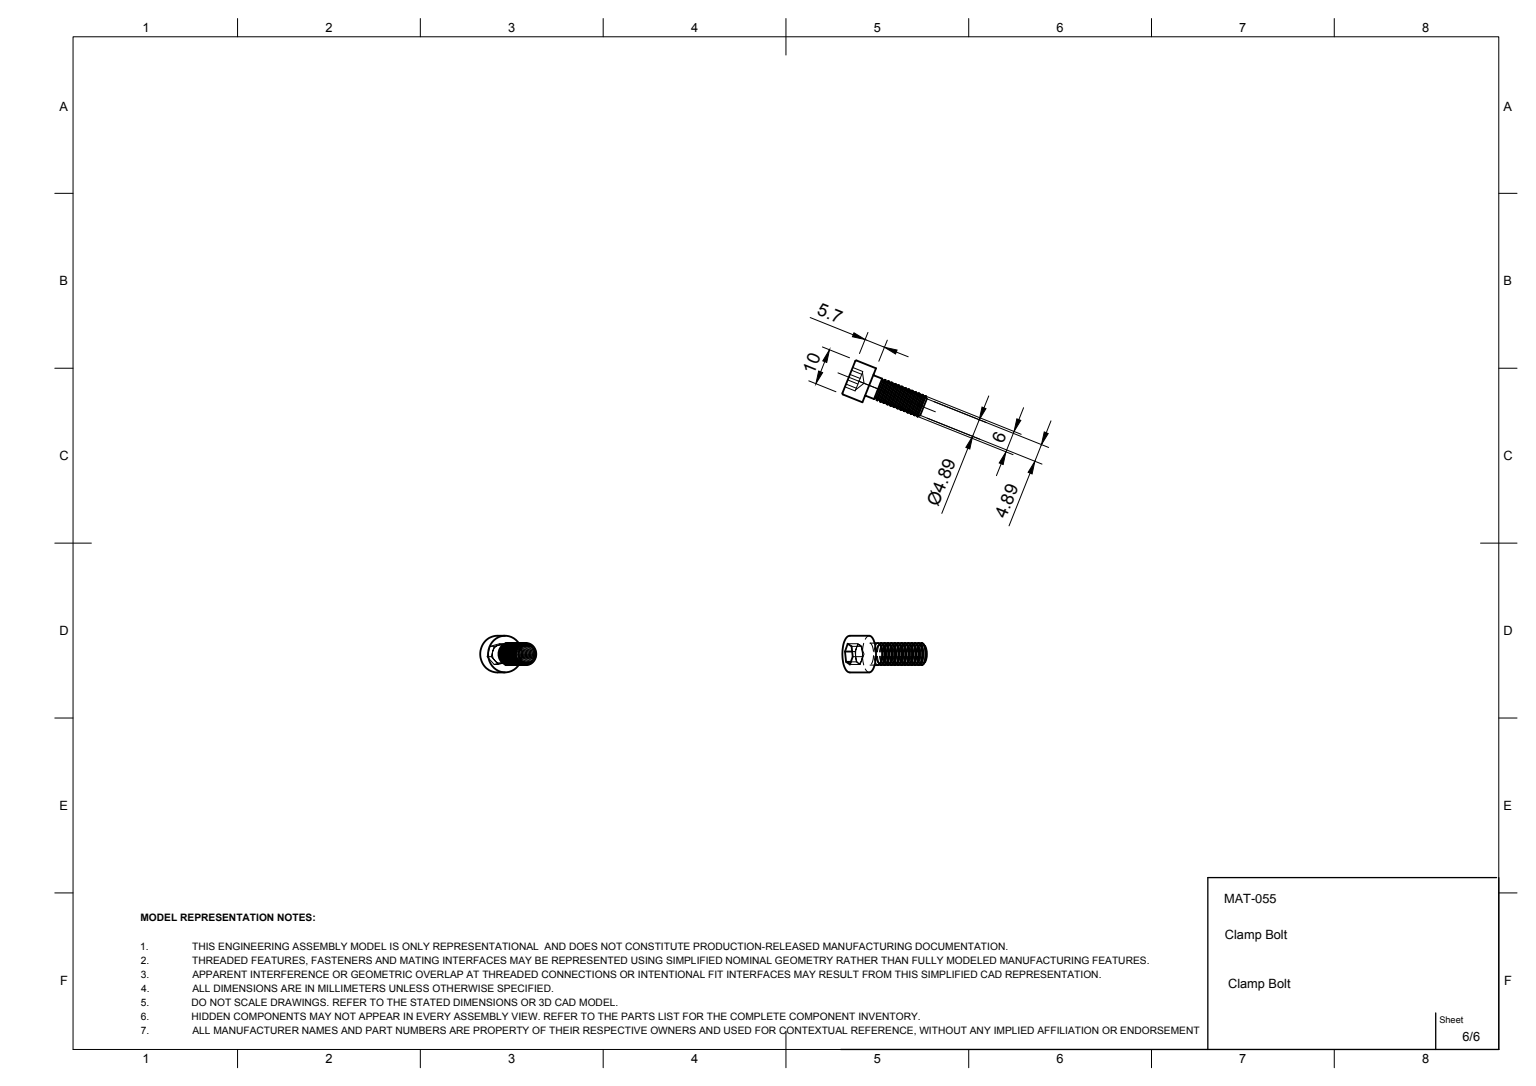
ISO-10303-21;
HEADER;
FILE_DESCRIPTION (('STEP AP214'),
    '1' );
FILE_NAME ('Clamp Bolt.step',
    '2026-10-30T09:41:00',
    ( '' ),
    ( '' ),
    'SwSTEP 2.0',
    'SolidWorks 2020',
    '' );
FILE_SCHEMA (( 'AUTOMOTIVE_DESIGN' ));
ENDSEC;

DATA;
#2=LINE ( 'NONE', #2744, #42488 ) ;
#10=FACE_OUTER_BOUND ( 'NONE', #7467, .T. ) ;
#27=AXIS2_PLACEMENT_3D ( 'NONE', #14609, #30094, #23021 ) ;
#30=LINE ( 'NONE', #27854, #4652 ) ;
#33=LINE ( 'NONE', #17589, #1125 ) ;
#38=DIRECTION ( 'NONE',  ( 0.9609149988134837450, -0.1028163501681639419, 0.2570431154366518145 ) ) ;
#58=DIRECTION ( 'NONE',  ( -0.000000000000000000, -0.9284778069183721172, -0.3713878862591650232 ) ) ;
#68=ORIENTED_EDGE ( 'NONE', *, *, #40399, .T. ) ;
#82=DIRECTION ( 'NONE',  ( 0.9609149988134837450, -0.1028163501681639419, 0.2570431154366518145 ) ) ;
#87=FACE_OUTER_BOUND ( 'NONE', #1657, .T. ) ;
#93=CARTESIAN_POINT ( 'NONE',  ( 71.02242295334774269, -99.02728775972636299, -55.91838671430374319 ) ) ;
#107=CARTESIAN_POINT ( 'NONE',  ( 69.36136150295220659, -60.18712133882883819, -34.17284023871924603 ) ) ;
#121=ORIENTED_EDGE ( 'NONE', *, *, #26803, .F. ) ;
#123=CIRCLE ( 'NONE', #28512, 2.445500000000004448 ) ;
#128=ORIENTED_EDGE ( 'NONE', *, *, #14994, .T. ) ;
#134=DIRECTION ( 'NONE',  ( -0.000000000000000000, -0.9284778069183718952, -0.3713878862591649677 ) ) ;
#135=CARTESIAN_POINT ( 'NONE',  ( 70.19189222814998175, -53.33815113939435548, -34.53808368179734600 ) ) ;
#167=CIRCLE ( 'NONE', #27232, 2.999999999999999556 ) ;
#169=AXIS2_PLACEMENT_3D ( 'NONE', #31050, #27866, #41779 ) ;
#179=EDGE_CURVE ( 'NONE', #39765, #40221, #19962, .T. ) ;
#191=CONICAL_SURFACE ( 'NONE', #23525, 2.999999999999999556, 0.9599310885968830309 ) ;
#193=VECTOR ( 'NONE', #10934, 1000.000000000000114 ) ;
#194=DIRECTION ( 'NONE',  ( -0.000000000000000000, -0.9284778069183721172, -0.3713878862591650232 ) ) ;
#216=EDGE_CURVE ( 'NONE', #33082, #17518, #26949, .T. ) ;
#219=VERTEX_POINT ( 'NONE', #5508 ) ;
#237=LINE ( 'NONE', #38306, #33556 ) ;
#238=EDGE_CURVE ( 'NONE', #18481, #11704, #33042, .T. ) ;
#251=DIRECTION ( 'NONE',  ( 0.2768435750659263284, 0.3568721902840676363, -0.8921882507333129819 ) ) ;
#252=CYLINDRICAL_SURFACE ( 'NONE', #41921, 3.000000000000001776 ) ;
#263=AXIS2_PLACEMENT_3D ( 'NONE', #1168, #7793, #17829 ) ;
#279=VERTEX_POINT ( 'NONE', #20785 ) ;
#280=AXIS2_PLACEMENT_3D ( 'NONE', #38645, #14273, #42543 ) ;
#302=LINE ( 'NONE', #3715, #30421 ) ;
#314=AXIS2_PLACEMENT_3D ( 'NONE', #35221, #3555, #37996 ) ;
#347=ORIENTED_EDGE ( 'NONE', *, *, #19251, .F. ) ;
#352=CARTESIAN_POINT ( 'NONE',  ( 67.84197459855160162, -60.15404070048191443, -37.99358876332483703 ) ) ;
#367=DIRECTION ( 'NONE',  ( -0.000000000000000000, -0.9284778069183718952, -0.3713878862591649677 ) ) ;
#384=CARTESIAN_POINT ( 'NONE',  ( 69.48536631248848039, -66.77523564985355620, -42.98127819198803934 ) ) ;
#406=CARTESIAN_POINT ( 'NONE',  ( 71.02242295334774269, -99.02728775972636299, -55.91838671430374319 ) ) ;
#416=CIRCLE ( 'NONE', #25919, 2.999999999999999556 ) ;
#429=DIRECTION ( 'NONE',  ( 1.387778780781445676E-17, -0.9284778069183720062, -0.3713878862591650232 ) ) ;
#435=FACE_OUTER_BOUND ( 'NONE', #25731, .T. ) ;
#454=DIRECTION ( 'NONE',  ( -0.2768435750659241079, -0.3568721902840695792, 0.8921882507333129819 ) ) ;
#482=DIRECTION ( 'NONE',  ( -0.2768435750659241079, -0.3568721902840695792, 0.8921882507333129819 ) ) ;
#487=DIRECTION ( 'NONE',  ( 0.9609149988134843001, -0.1028163501681632064, 0.2570431154366505933 ) ) ;
#495=EDGE_CURVE ( 'NONE', #29216, #38926, #30, .T. ) ;
#519=VECTOR ( 'NONE', #2199, 999.9999999999998863 ) ;
#545=ORIENTED_EDGE ( 'NONE', *, *, #32038, .F. ) ;
#572=AXIS2_PLACEMENT_3D ( 'NONE', #28197, #18381, #24548 ) ;
#587=EDGE_CURVE ( 'NONE', #3470, #34725, #44742, .T. ) ;
#591=DIRECTION ( 'NONE',  ( -0.000000000000000000, -0.9284778069183721172, -0.3713878862591650232 ) ) ;
#628=ORIENTED_EDGE ( 'NONE', *, *, #2447, .F. ) ;
#652=DIRECTION ( 'NONE',  ( 0.000000000000000000, 0.9284778069183720062, 0.3713878862591650232 ) ) ;
#663=ORIENTED_EDGE ( 'NONE', *, *, #32365, .T. ) ;
#730=ORIENTED_EDGE ( 'NONE', *, *, #26390, .T. ) ;
#731=AXIS2_PLACEMENT_3D ( 'NONE', #25829, #15568, #36529 ) ;
#769=LINE ( 'NONE', #29271, #10675 ) ;
#793=DIRECTION ( 'NONE',  ( -0.7871354856660162103, -0.4483307682966942709, -0.4235767337848251879 ) ) ;
#796=EDGE_CURVE ( 'NONE', #20803, #26292, #18485, .T. ) ;
#800=DIRECTION ( 'NONE',  ( 0.9609149988134837450, -0.1028163501681639419, 0.2570431154366518145 ) ) ;
#825=CONICAL_SURFACE ( 'NONE', #24153, 2.999999999999999556, 0.9599310885968830309 ) ;
#838=CARTESIAN_POINT ( 'NONE',  ( 70.19189222814998175, -62.26243369865490251, -38.10776559704283528 ) ) ;
#860=DIRECTION ( 'NONE',  ( -0.000000000000000000, -0.9284778069183718952, -0.3713878862591649677 ) ) ;
#871=FACE_OUTER_BOUND ( 'NONE', #3620, .T. ) ;
#876=LINE ( 'NONE', #14795, #14624 ) ;
#877=CARTESIAN_POINT ( 'NONE',  ( 70.19189222814998175, -59.83749578782295941, -37.13779888561150244 ) ) ;
#907=LINE ( 'NONE', #38753, #23410 ) ;
#909=AXIS2_PLACEMENT_3D ( 'NONE', #40106, #12526, #26200 ) ;
#910=DIRECTION ( 'NONE',  ( -0.000000000000000000, -0.9284778069183721172, -0.3713878862591650232 ) ) ;
#935=EDGE_CURVE ( 'NONE', #32198, #39653, #29454, .T. ) ;
#964=ORIENTED_EDGE ( 'NONE', *, *, #27844, .T. ) ;
#989=AXIS2_PLACEMENT_3D ( 'NONE', #41662, #38211, #6989 ) ;
#993=ORIENTED_EDGE ( 'NONE', *, *, #15751, .F. ) ;
#1002=ORIENTED_EDGE ( 'NONE', *, *, #1925, .F. ) ;
#1047=EDGE_CURVE ( 'NONE', #6949, #28070, #36732, .T. ) ;
#1065=ADVANCED_FACE ( 'NONE', ( #27355 ), #14883, .T. ) ;
#1068=AXIS2_PLACEMENT_3D ( 'NONE', #35389, #28345, #42258 ) ;
#1098=DIRECTION ( 'NONE',  ( -0.000000000000000000, -0.9284778069183720062, -0.3713878862591650232 ) ) ;
#1101=ORIENTED_EDGE ( 'NONE', *, *, #11741, .F. ) ;
#1112=EDGE_CURVE ( 'NONE', #13294, #44431, #30929, .T. ) ;
#1113=CARTESIAN_POINT ( 'NONE',  ( 73.01241679510815175, -68.13509210538408922, -39.58160742654554554 ) ) ;
#1125=VECTOR ( 'NONE', #32153, 1000.000000000000227 ) ;
#1156=CIRCLE ( 'NONE', #35346, 2.999999999999999556 ) ;
#1168=CARTESIAN_POINT ( 'NONE',  ( 70.19189222814998175, -67.83330054016514055, -40.33609291459782753 ) ) ;
#1187=AXIS2_PLACEMENT_3D ( 'NONE', #31508, #41577, #10337 ) ;
#1210=CARTESIAN_POINT ( 'NONE',  ( 72.54180985774836188, -52.30061520688905574, -33.39389990939168484 ) ) ;
#1216=AXIS2_PLACEMENT_3D ( 'NONE', #18061, #29000, #39027 ) ;
#1227=AXIS2_PLACEMENT_3D ( 'NONE', #27267, #34086, #17229 ) ;
#1232=EDGE_CURVE ( 'NONE', #1783, #34215, #3962, .T. ) ;
#1241=AXIS2_PLACEMENT_3D ( 'NONE', #14999, #18647, #4950 ) ;
#1250=VECTOR ( 'NONE', #33138, 1000.000000000000000 ) ;
#1264=DIRECTION ( 'NONE',  ( -0.7871354856660162103, -0.4483307682966942709, -0.4235767337848251879 ) ) ;
#1280=DIRECTION ( 'NONE',  ( -0.7871354856660162103, -0.4483307682966942709, -0.4235767337848251879 ) ) ;
#1303=ORIENTED_EDGE ( 'NONE', *, *, #23992, .F. ) ;
#1306=ORIENTED_EDGE ( 'NONE', *, *, #37165, .T. ) ;
#1309=DIRECTION ( 'NONE',  ( -0.2768435750659241079, -0.3568721902840695792, 0.8921882507333129819 ) ) ;
#1349=EDGE_CURVE ( 'NONE', #34283, #41097, #1533, .T. ) ;
#1365=ADVANCED_FACE ( 'NONE', ( #21395 ), #4280, .T. ) ;
#1388=DIRECTION ( 'NONE',  ( 0.9609149988134839671, -0.1028163501681660097, 0.2570431154366504822 ) ) ;
#1401=ORIENTED_EDGE ( 'NONE', *, *, #11163, .F. ) ;
#1418=CARTESIAN_POINT ( 'NONE',  ( 70.19189222814998175, -60.76597359474132531, -37.50918677187066663 ) ) ;
#1435=ORIENTED_EDGE ( 'NONE', *, *, #6611, .F. ) ;
#1437=CARTESIAN_POINT ( 'NONE',  ( 67.37136766119182596, -67.53150897494617766, -41.09057840265009531 ) ) ;
#1444=VERTEX_POINT ( 'NONE', #7933 ) ;
#1453=DIRECTION ( 'NONE',  ( 0.000000000000000000, 0.9284778069183720062, 0.3713878862591650232 ) ) ;
#1526=DIRECTION ( 'NONE',  ( 0.000000000000000000, 0.9284778069183721172, 0.3713878862591650232 ) ) ;
#1533=LINE ( 'NONE', #39627, #5454 ) ;
#1552=ORIENTED_EDGE ( 'NONE', *, *, #28698, .T. ) ;
#1561=CIRCLE ( 'NONE', #20499, 2.445500000000004448 ) ;
#1577=ORIENTED_EDGE ( 'NONE', *, *, #36322, .F. ) ;
#1583=EDGE_CURVE ( 'NONE', #44494, #13382, #6190, .T. ) ;
#1584=DIRECTION ( 'NONE',  ( -0.000000000000000000, -0.9284778069183721172, -0.3713878862591650232 ) ) ;
#1610=CARTESIAN_POINT ( 'NONE',  ( 70.19189222814998175, -50.19222220871606766, -33.27972307567368659 ) ) ;
#1622=EDGE_CURVE ( 'NONE', #14508, #21214, #22199, .T. ) ;
#1624=DIRECTION ( 'NONE',  ( 0.9609149988134837450, -0.1028163501681639419, 0.2570431154366518145 ) ) ;
#1657=EDGE_LOOP ( 'NONE', ( #10871, #34682, #25094, #19004 ) ) ;
#1665=VERTEX_POINT ( 'NONE', #26616 ) ;
#1666=VECTOR ( 'NONE', #17254, 1000.000000000000000 ) ;
#1693=CARTESIAN_POINT ( 'NONE',  ( 70.19189222814998175, -56.69156685714467159, -35.87943827948784303 ) ) ;
#1720=CONICAL_SURFACE ( 'NONE', #33641, 2.999999999999999556, 0.9599310885968830309 ) ;
#1732=ORIENTED_EDGE ( 'NONE', *, *, #30164, .F. ) ;
#1734=CONICAL_SURFACE ( 'NONE', #37413, 2.445500000000004448, 0.9599310885968757034 ) ;
#1750=CARTESIAN_POINT ( 'NONE',  ( 73.07463722459043254, -54.57507799681722105, -34.13834222174655508 ) ) ;
#1762=VERTEX_POINT ( 'NONE', #27971 ) ;
#1772=AXIS2_PLACEMENT_3D ( 'NONE', #30439, #24060, #27478 ) ;
#1780=DIRECTION ( 'NONE',  ( -0.2768435750659241079, -0.3568721902840695792, 0.8921882507333129819 ) ) ;
#1783=VERTEX_POINT ( 'NONE', #41440 ) ;
#1832=CARTESIAN_POINT ( 'NONE',  ( 70.19189222814998175, -53.33815113939435548, -34.53808368179734600 ) ) ;
#1853=ORIENTED_EDGE ( 'NONE', *, *, #33091, .F. ) ;
#1854=ORIENTED_EDGE ( 'NONE', *, *, #10017, .T. ) ;
#1858=DIRECTION ( 'NONE',  ( -0.000000000000000000, -0.9284778069183721172, -0.3713878862591650232 ) ) ;
#1860=CIRCLE ( 'NONE', #27379, 2.541999999999999371 ) ;
#1861=DIRECTION ( 'NONE',  ( 0.9609149988134837450, -0.1028163501681639419, 0.2570431154366518145 ) ) ;
#1898=ORIENTED_EDGE ( 'NONE', *, *, #39518, .F. ) ;
#1899=ADVANCED_FACE ( 'NONE', ( #34121 ), #28031, .T. ) ;
#1919=EDGE_CURVE ( 'NONE', #33992, #25917, #8371, .T. ) ;
#1925=EDGE_CURVE ( 'NONE', #40221, #22169, #36765, .T. ) ;
#1926=ORIENTED_EDGE ( 'NONE', *, *, #2248, .F. ) ;
#1937=ORIENTED_EDGE ( 'NONE', *, *, #35623, .T. ) ;
#1942=CIRCLE ( 'NONE', #7033, 2.999999999999999556 ) ;
#1946=DIRECTION ( 'NONE',  ( -0.000000000000000000, -0.9284778069183721172, -0.3713878862591650232 ) ) ;
#1962=AXIS2_PLACEMENT_3D ( 'NONE', #35730, #25036, #28690 ) ;
#1974=CIRCLE ( 'NONE', #23849, 2.999999999999999556 ) ;
#2036=LINE ( 'NONE', #30314, #37177 ) ;
#2059=FACE_OUTER_BOUND ( 'NONE', #24766, .T. ) ;
#2074=EDGE_LOOP ( 'NONE', ( #5365, #14211, #39192, #1577, #22410, #32120 ) ) ;
#2105=DIRECTION ( 'NONE',  ( -0.000000000000000000, -0.9284778069183721172, -0.3713878862591650232 ) ) ;
#2118=CIRCLE ( 'NONE', #36346, 2.999999999999999556 ) ;
#2119=LINE ( 'NONE', #6857, #35006 ) ;
#2129=CARTESIAN_POINT ( 'NONE',  ( 70.19189222814998175, -59.11650476797663600, -36.84940499091918298 ) ) ;
#2154=CIRCLE ( 'NONE', #26946, 4.999999999999998224 ) ;
#2158=EDGE_CURVE ( 'NONE', #13382, #35800, #29749, .T. ) ;
#2180=AXIS2_PLACEMENT_3D ( 'NONE', #22807, #19390, #12787 ) ;
#2199=DIRECTION ( 'NONE',  ( -0.7871354856660162103, -0.4483307682966942709, -0.4235767337848251879 ) ) ;
#2210=ORIENTED_EDGE ( 'NONE', *, *, #7604, .T. ) ;
#2226=AXIS2_PLACEMENT_3D ( 'NONE', #31900, #39655, #15484 ) ;
#2248=EDGE_CURVE ( 'NONE', #219, #6975, #23691, .T. ) ;
#2254=CIRCLE ( 'NONE', #26288, 2.999999999999999556 ) ;
#2291=VECTOR ( 'NONE', #33970, 999.9999999999998863 ) ;
#2301=EDGE_CURVE ( 'NONE', #39549, #1444, #33117, .T. ) ;
#2315=DIRECTION ( 'NONE',  ( 0.9609149988134837450, -0.1028163501681639419, 0.2570431154366518145 ) ) ;
#2317=DIRECTION ( 'NONE',  ( -0.000000000000000000, -0.9284778069183721172, -0.3713878862591650232 ) ) ;
#2325=EDGE_LOOP ( 'NONE', ( #33811, #7565, #42276, #17085, #17615 ) ) ;
#2361=VERTEX_POINT ( 'NONE', #31102 ) ;
#2387=ORIENTED_EDGE ( 'NONE', *, *, #10017, .F. ) ;
#2395=DIRECTION ( 'NONE',  ( -0.000000000000000000, -0.9284778069183718952, -0.3713878862591649677 ) ) ;
#2396=LINE ( 'NONE', #31119, #17256 ) ;
#2421=CARTESIAN_POINT ( 'NONE',  ( 70.19189222814998175, -50.76020450571126474, -33.50691401458669105 ) ) ;
#2428=DIRECTION ( 'NONE',  ( -0.2768435750659263839, -0.3568721902840676363, 0.8921882507333129819 ) ) ;
#2447=EDGE_CURVE ( 'NONE', #41822, #12164, #16995, .T. ) ;
#2456=ORIENTED_EDGE ( 'NONE', *, *, #43751, .F. ) ;
#2475=LINE ( 'NONE', #16400, #43937 ) ;
#2516=DIRECTION ( 'NONE',  ( 0.2768435750659241079, 0.3568721902840695792, -0.8921882507333129819 ) ) ;
#2537=ORIENTED_EDGE ( 'NONE', *, *, #43419, .T. ) ;
#2553=CARTESIAN_POINT ( 'NONE',  ( 70.19189222814998175, -55.40259354030312267, -35.36385344588251911 ) ) ;
#2555=AXIS2_PLACEMENT_3D ( 'NONE', #12768, #9114, #15276 ) ;
#2559=EDGE_CURVE ( 'NONE', #20329, #10520, #3509, .T. ) ;
#2568=CARTESIAN_POINT ( 'NONE',  ( 67.30914723170953096, -56.74361331656334784, -36.79476457314395788 ) ) ;
#2571=DIRECTION ( 'NONE',  ( -0.7871354856660162103, -0.4483307682966942709, -0.4235767337848251879 ) ) ;
#2594=DIRECTION ( 'NONE',  ( -0.000000000000000000, -0.9284778069183721172, -0.3713878862591650232 ) ) ;
#2597=ORIENTED_EDGE ( 'NONE', *, *, #22814, .T. ) ;
#2641=ORIENTED_EDGE ( 'NONE', *, *, #30471, .T. ) ;
#2678=CONICAL_SURFACE ( 'NONE', #7079, 2.999999999999999556, 0.9599310885968830309 ) ;
#2680=VERTEX_POINT ( 'NONE', #25554 ) ;
#2686=ORIENTED_EDGE ( 'NONE', *, *, #6157, .T. ) ;
#2690=ORIENTED_EDGE ( 'NONE', *, *, #24599, .T. ) ;
#2709=ORIENTED_EDGE ( 'NONE', *, *, #14877, .F. ) ;
#2744=CARTESIAN_POINT ( 'NONE',  ( 72.54180985774836188, -62.51387108299115170, -37.47916665824249804 ) ) ;
#2761=EDGE_CURVE ( 'NONE', #36562, #29748, #3265, .T. ) ;
#2764=EDGE_CURVE ( 'NONE', #19894, #21045, #30863, .T. ) ;
#2777=CIRCLE ( 'NONE', #23195, 2.999999999999999556 ) ;
#2812=ORIENTED_EDGE ( 'NONE', *, *, #4709, .F. ) ;
#2826=ORIENTED_EDGE ( 'NONE', *, *, #14877, .T. ) ;
#2827=DIRECTION ( 'NONE',  ( 0.000000000000000000, 0.9284778069183720062, 0.3713878862591650232 ) ) ;
#2839=CARTESIAN_POINT ( 'NONE',  ( 70.19189222814998175, -100.0979043305785581, -53.24182196210380624 ) ) ;
#2872=ORIENTED_EDGE ( 'NONE', *, *, #44296, .T. ) ;
#2911=DIRECTION ( 'NONE',  ( 0.7202110682883375858, 0.2576522076061144029, -0.6441361323747234469 ) ) ;
#2917=DIRECTION ( 'NONE',  ( -0.000000000000000000, -0.9284778069183721172, -0.3713878862591650232 ) ) ;
#2964=VERTEX_POINT ( 'NONE', #34918 ) ;
#2999=DIRECTION ( 'NONE',  ( -0.000000000000000000, -0.9284778069183721172, -0.3713878862591650232 ) ) ;
#3005=CIRCLE ( 'NONE', #32124, 2.999999999999999556 ) ;
#3006=DIRECTION ( 'NONE',  ( -0.000000000000000000, -0.9284778069183718952, -0.3713878862591649677 ) ) ;
#3022=EDGE_CURVE ( 'NONE', #42672, #1762, #4029, .T. ) ;
#3028=EDGE_CURVE ( 'NONE', #20614, #29197, #33873, .T. ) ;
#3034=ORIENTED_EDGE ( 'NONE', *, *, #26998, .T. ) ;
#3035=CARTESIAN_POINT ( 'NONE',  ( 70.19189222814998175, -57.25954915413987578, -36.10662921840084749 ) ) ;
#3050=ORIENTED_EDGE ( 'NONE', *, *, #25617, .T. ) ;
#3056=CARTESIAN_POINT ( 'NONE',  ( 70.19189222814998175, -61.33395589173652951, -37.73637771078367109 ) ) ;
#3080=CYLINDRICAL_SURFACE ( 'NONE', #38052, 3.000000000000001776 ) ;
#3082=CARTESIAN_POINT ( 'NONE',  ( 70.19189222814998175, -57.62004466406304459, -36.25082616574700722 ) ) ;
#3104=AXIS2_PLACEMENT_3D ( 'NONE', #28209, #4242, #14515 ) ;
#3123=DIRECTION ( 'NONE',  ( 0.9609149988134843001, -0.1028163501681632064, 0.2570431154366505933 ) ) ;
#3126=VERTEX_POINT ( 'NONE', #18070 ) ;
#3129=DIRECTION ( 'NONE',  ( -0.000000000000000000, -0.9284778069183720062, -0.3713878862591650232 ) ) ;
#3140=EDGE_CURVE ( 'NONE', #31689, #36176, #21490, .T. ) ;
#3153=CIRCLE ( 'NONE', #30069, 2.999999999999999556 ) ;
#3205=CARTESIAN_POINT ( 'NONE',  ( 70.19189222814998175, -50.76020450571126474, -33.50691401458669105 ) ) ;
#3209=DIRECTION ( 'NONE',  ( 0.9609149988134837450, -0.1028163501681639419, 0.2570431154366518145 ) ) ;
#3228=CARTESIAN_POINT ( 'NONE',  ( 67.30914723170953096, -57.87957791055376333, -37.24914645096997390 ) ) ;
#3248=CARTESIAN_POINT ( 'NONE',  ( 70.19189222814998175, -61.90193818873174791, -37.96356864969668266 ) ) ;
#3250=CARTESIAN_POINT ( 'NONE',  ( 67.84197459855160162, -61.08251850740028033, -38.36497664958400122 ) ) ;
#3265=LINE ( 'NONE', #6918, #11338 ) ;
#3275=EDGE_CURVE ( 'NONE', #32855, #40329, #32189, .T. ) ;
#3277=EDGE_LOOP ( 'NONE', ( #17579, #9420, #5051, #7378, #14820 ) ) ;
#3278=CARTESIAN_POINT ( 'NONE',  ( 70.19189222814998175, -54.47411573338475677, -34.99246555962335492 ) ) ;
#3288=VECTOR ( 'NONE', #34511, 999.9999999999998863 ) ;
#3295=ORIENTED_EDGE ( 'NONE', *, *, #22804, .F. ) ;
#3329=FACE_OUTER_BOUND ( 'NONE', #11678, .T. ) ;
#3352=DIRECTION ( 'NONE',  ( -0.9609149988134838560, 0.1028163501681644970, -0.2570431154366519810 ) ) ;
#3367=DIRECTION ( 'NONE',  ( 0.9609149988134837450, -0.1028163501681639419, 0.2570431154366518145 ) ) ;
#3391=ORIENTED_EDGE ( 'NONE', *, *, #4145, .F. ) ;
#3394=DIRECTION ( 'NONE',  ( -0.000000000000000000, -0.9284778069183718952, -0.3713878862591649677 ) ) ;
#3397=EDGE_CURVE ( 'NONE', #20803, #8943, #29560, .T. ) ;
#3400=DIRECTION ( 'NONE',  ( 0.9609149988134837450, -0.1028163501681639419, 0.2570431154366518145 ) ) ;
#3408=ORIENTED_EDGE ( 'NONE', *, *, #4467, .T. ) ;
#3423=CARTESIAN_POINT ( 'NONE',  ( 71.57611010347959279, -98.31354337915821873, -57.70276321577036782 ) ) ;
#3431=DIRECTION ( 'NONE',  ( -0.9609149988134837450, 0.1028163501681639419, -0.2570431154366518145 ) ) ;
#3433=ORIENTED_EDGE ( 'NONE', *, *, #10899, .F. ) ;
#3470=VERTEX_POINT ( 'NONE', #6309 ) ;
#3493=ORIENTED_EDGE ( 'NONE', *, *, #37007, .T. ) ;
#3509=LINE ( 'NONE', #93, #21514 ) ;
#3549=DIRECTION ( 'NONE',  ( 0.9609149988134837450, -0.1028163501681639419, 0.2570431154366518145 ) ) ;
#3550=EDGE_CURVE ( 'NONE', #31200, #33021, #416, .T. ) ;
#3555=DIRECTION ( 'NONE',  ( -0.000000000000000000, -0.9284778069183718952, -0.3713878862591649677 ) ) ;
#3559=DIRECTION ( 'NONE',  ( 0.9609149988134843001, -0.1028163501681632064, 0.2570431154366505933 ) ) ;
#3581=EDGE_CURVE ( 'NONE', #39890, #16741, #33183, .T. ) ;
#3589=ORIENTED_EDGE ( 'NONE', *, *, #34569, .T. ) ;
#3599=ORIENTED_EDGE ( 'NONE', *, *, #39791, .F. ) ;
#3620=EDGE_LOOP ( 'NONE', ( #6263, #33817, #3948, #26256, #121 ) ) ;
#3659=ORIENTED_EDGE ( 'NONE', *, *, #18597, .F. ) ;
#3660=AXIS2_PLACEMENT_3D ( 'NONE', #31392, #26864, #9537 ) ;
#3667=FACE_OUTER_BOUND ( 'NONE', #38630, .T. ) ;
#3675=ORIENTED_EDGE ( 'NONE', *, *, #30870, .F. ) ;
#3701=VECTOR ( 'NONE', #43009, 1000.000000000000227 ) ;
#3705=EDGE_LOOP ( 'NONE', ( #40200, #22267, #41392, #19038, #4373 ) ) ;
#3715=CARTESIAN_POINT ( 'NONE',  ( 69.48536631248848039, -66.77523564985355620, -42.98127819198803934 ) ) ;
#3751=DIRECTION ( 'NONE',  ( 0.9609149988134837450, -0.1028163501681639419, 0.2570431154366518145 ) ) ;
#3754=VERTEX_POINT ( 'NONE', #36570 ) ;
#3775=FACE_OUTER_BOUND ( 'NONE', #42003, .T. ) ;
#3791=CARTESIAN_POINT ( 'NONE',  ( 70.89841814381148311, -68.89136543047671069, -37.69090763720760151 ) ) ;
#3799=EDGE_LOOP ( 'NONE', ( #29590, #18190, #29958, #27592, #31507 ) ) ;
#3802=EDGE_CURVE ( 'NONE', #44494, #30068, #22226, .T. ) ;
#3810=ADVANCED_FACE ( 'NONE', ( #12427 ), #22269, .T. ) ;
#3822=CARTESIAN_POINT ( 'NONE',  ( 70.19189222814998175, -51.48119552555760947, -33.79530790927901052 ) ) ;
#3852=DIRECTION ( 'NONE',  ( -0.9705985873829334754, -0.08939452397200675637, 0.2234882575306194330 ) ) ;
#3855=ADVANCED_FACE ( 'NONE', ( #37245 ), #36081, .T. ) ;
#3856=ORIENTED_EDGE ( 'NONE', *, *, #4513, .T. ) ;
#3874=ORIENTED_EDGE ( 'NONE', *, *, #20558, .T. ) ;
#3879=AXIS2_PLACEMENT_3D ( 'NONE', #40112, #8876, #29850 ) ;
#3903=CARTESIAN_POINT ( 'NONE',  ( 70.19189222814998175, -51.12070001563444066, -33.65111096193285078 ) ) ;
#3915=ORIENTED_EDGE ( 'NONE', *, *, #36564, .F. ) ;
#3916=CONICAL_SURFACE ( 'NONE', #29405, 2.999999999999999556, 0.9599310885968830309 ) ;
#3931=EDGE_CURVE ( 'NONE', #29125, #30068, #23009, .T. ) ;
#3948=ORIENTED_EDGE ( 'NONE', *, *, #26611, .T. ) ;
#3955=ORIENTED_EDGE ( 'NONE', *, *, #34508, .T. ) ;
#3962=CIRCLE ( 'NONE', #17081, 3.249999999999996003 ) ;
#3974=DIRECTION ( 'NONE',  ( 0.9609149988134837450, -0.1028163501681639419, 0.2570431154366518145 ) ) ;
#3988=AXIS2_PLACEMENT_3D ( 'NONE', #13113, #37490, #9459 ) ;
#4000=CARTESIAN_POINT ( 'NONE',  ( 70.19189222814998175, -52.40967333247598248, -34.16669579553818181 ) ) ;
#4001=CARTESIAN_POINT ( 'NONE',  ( 67.30914723170953096, -61.38600235115519865, -38.65170400443977883 ) ) ;
#4019=DIRECTION ( 'NONE',  ( 0.9609149988134834119, -0.1028163501681649411, 0.2570431154366530913 ) ) ;
#4027=VERTEX_POINT ( 'NONE', #6017 ) ;
#4029=CIRCLE ( 'NONE', #25876, 2.999999999999999556 ) ;
#4063=DIRECTION ( 'NONE',  ( 0.9609149988134837450, -0.1028163501681639419, 0.2570431154366518145 ) ) ;
#4083=DIRECTION ( 'NONE',  ( -0.000000000000000000, -0.9284778069183718952, -0.3713878862591649677 ) ) ;
#4086=ORIENTED_EDGE ( 'NONE', *, *, #30471, .F. ) ;
#4087=ADVANCED_FACE ( 'NONE', ( #6931 ), #38263, .T. ) ;
#4105=ADVANCED_FACE ( 'NONE', ( #20838 ), #14981, .T. ) ;
#4108=DIRECTION ( 'NONE',  ( -0.000000000000000000, -0.9284778069183721172, -0.3713878862591650232 ) ) ;
#4119=CYLINDRICAL_SURFACE ( 'NONE', #16259, 3.000000000000001776 ) ;
#4134=FACE_OUTER_BOUND ( 'NONE', #28235, .T. ) ;
#4143=VECTOR ( 'NONE', #793, 999.9999999999998863 ) ;
#4145=EDGE_CURVE ( 'NONE', #13251, #31200, #37560, .T. ) ;
#4159=( GEOMETRIC_REPRESENTATION_CONTEXT ( 3 ) GLOBAL_UNCERTAINTY_ASSIGNED_CONTEXT ( ( #15884 ) ) GLOBAL_UNIT_ASSIGNED_CONTEXT ( ( #23883, #27067, #41211 ) ) REPRESENTATION_CONTEXT ( 'NONE', 'WORKASPACE' ) );
#4171=CIRCLE ( 'NONE', #18012, 2.999999999999999556 ) ;
#4180=CARTESIAN_POINT ( 'NONE',  ( 72.54180985774836188, -59.72843766223603268, -36.36500299946500547 ) ) ;
#4194=DIRECTION ( 'NONE',  ( -0.000000000000000000, -0.9284778069183721172, -0.3713878862591650232 ) ) ;
#4202=CARTESIAN_POINT ( 'NONE',  ( 69.36136150295220659, -63.69354577943025930, -35.57539779218904386 ) ) ;
#4219=CARTESIAN_POINT ( 'NONE',  ( 70.19189222814998175, -52.40967333247598248, -34.16669579553818181 ) ) ;
#4242=DIRECTION ( 'NONE',  ( -0.000000000000000000, -0.9284778069183720062, -0.3713878862591650232 ) ) ;
#4255=ORIENTED_EDGE ( 'NONE', *, *, #9672, .F. ) ;
#4267=ORIENTED_EDGE ( 'NONE', *, *, #38622, .F. ) ;
#4275=DIRECTION ( 'NONE',  ( -0.000000000000000000, -0.9284778069183721172, -0.3713878862591650232 ) ) ;
#4280=PLANE ( 'NONE',  #38204 ) ;
#4287=CARTESIAN_POINT ( 'NONE',  ( 70.19189222814998175, -58.54852247098141049, -36.62221405200617141 ) ) ;
#4294=LINE ( 'NONE', #22312, #24049 ) ;
#4296=ORIENTED_EDGE ( 'NONE', *, *, #7655, .F. ) ;
#4309=EDGE_CURVE ( 'NONE', #1665, #10336, #14441, .T. ) ;
#4311=DIRECTION ( 'NONE',  ( 0.9609149988134843001, -0.1028163501681632064, 0.2570431154366505933 ) ) ;
#4327=ORIENTED_EDGE ( 'NONE', *, *, #25222, .T. ) ;
#4331=CIRCLE ( 'NONE', #41413, 2.999999999999999556 ) ;
#4333=CARTESIAN_POINT ( 'NONE',  ( 73.07463722459043254, -59.42495381848112856, -36.07827564460922787 ) ) ;
#4363=VERTEX_POINT ( 'NONE', #42261 ) ;
#4373=ORIENTED_EDGE ( 'NONE', *, *, #34780, .T. ) ;
#4376=VECTOR ( 'NONE', #43012, 1000.000000000000114 ) ;
#4381=CIRCLE ( 'NONE', #17532, 2.999999999999999556 ) ;
#4387=VERTEX_POINT ( 'NONE', #11250 ) ;
#4403=DIRECTION ( 'NONE',  ( 0.000000000000000000, 0.9284778069183721172, 0.3713878862591650232 ) ) ;
#4410=DIRECTION ( 'NONE',  ( -0.000000000000000000, -0.9284778069183720062, -0.3713878862591650232 ) ) ;
#4413=CIRCLE ( 'NONE', #34288, 2.999999999999999556 ) ;
#4419=CARTESIAN_POINT ( 'NONE',  ( 72.54180985774836188, -58.79995985531765967, -35.99361511320584128 ) ) ;
#4420=DIRECTION ( 'NONE',  ( 0.9609149988134837450, -0.1028163501681639419, 0.2570431154366518145 ) ) ;
#4446=VECTOR ( 'NONE', #37878, 1000.000000000000114 ) ;
#4460=PLANE ( 'NONE',  #572 ) ;
#4467=EDGE_CURVE ( 'NONE', #12877, #16491, #44160, .T. ) ;
#4480=DIRECTION ( 'NONE',  ( -0.000000000000000000, -0.9284778069183721172, -0.3713878862591650232 ) ) ;
#4513=EDGE_CURVE ( 'NONE', #26262, #37456, #26892, .T. ) ;
#4529=ORIENTED_EDGE ( 'NONE', *, *, #12554, .F. ) ;
#4564=CARTESIAN_POINT ( 'NONE',  ( 67.30914723170953096, -58.80805571747214344, -37.62053433722914519 ) ) ;
#4583=CARTESIAN_POINT ( 'NONE',  ( 67.84197459855160162, -57.36860727972680252, -36.87942510454734446 ) ) ;
#4589=ORIENTED_EDGE ( 'NONE', *, *, #24222, .F. ) ;
#4596=PRODUCT_DEFINITION_CONTEXT ( 'detailed design', #40213, 'design' ) ;
#4616=VECTOR ( 'NONE', #15882, 1000.000000000000227 ) ;
#4627=VECTOR ( 'NONE', #20845, 999.9999999999998863 ) ;
#4633=DIRECTION ( 'NONE',  ( 0.9609149988134837450, -0.1028163501681639419, 0.2570431154366518145 ) ) ;
#4652=VECTOR ( 'NONE', #27634, 1000.000000000000227 ) ;
#4677=LINE ( 'NONE', #18598, #17313 ) ;
#4682=ORIENTED_EDGE ( 'NONE', *, *, #38681, .T. ) ;
#4696=CARTESIAN_POINT ( 'NONE',  ( 73.01241679510815175, -68.13509210538408922, -39.58160742654554554 ) ) ;
#4709=EDGE_CURVE ( 'NONE', #15070, #23958, #36857, .T. ) ;
#4717=ADVANCED_FACE ( 'NONE', ( #41964 ), #42858, .T. ) ;
#4718=AXIS2_PLACEMENT_3D ( 'NONE', #14274, #11305, #25214 ) ;
#4729=LINE ( 'NONE', #5847, #519 ) ;
#4731=FACE_OUTER_BOUND ( 'NONE', #29352, .T. ) ;
#4768=ORIENTED_EDGE ( 'NONE', *, *, #41411, .F. ) ;
#4774=EDGE_CURVE ( 'NONE', #44682, #27626, #39435, .T. ) ;
#4778=PLANE ( 'NONE',  #19126 ) ;
#4780=ORIENTED_EDGE ( 'NONE', *, *, #43691, .T. ) ;
#4806=DIRECTION ( 'NONE',  ( -0.000000000000000000, -0.9284778069183721172, -0.3713878862591650232 ) ) ;
#4821=VERTEX_POINT ( 'NONE', #42412 ) ;
#4839=CONICAL_SURFACE ( 'NONE', #25981, 2.999999999999999556, 0.9599310885968830309 ) ;
#4852=ORIENTED_EDGE ( 'NONE', *, *, #44578, .F. ) ;
#4888=AXIS2_PLACEMENT_3D ( 'NONE', #2421, #6531, #37304 ) ;
#4889=DIRECTION ( 'NONE',  ( -0.9609149988134837450, 0.1028163501681639419, -0.2570431154366518145 ) ) ;
#4907=CARTESIAN_POINT ( 'NONE',  ( 69.51487126532624927, -51.06495315005575719, -31.09787670850536756 ) ) ;
#4948=CARTESIAN_POINT ( 'NONE',  ( 70.19189222814998175, -70.34019061884472990, -41.33884020749756871 ) ) ;
#4950=DIRECTION ( 'NONE',  ( 0.9609149988134837450, -0.1028163501681639419, 0.2570431154366518145 ) ) ;
#4955=CARTESIAN_POINT ( 'NONE',  ( 70.19189222814998175, -65.04786711941001442, -39.22192925582032785 ) ) ;
#4956=EDGE_CURVE ( 'NONE', #8943, #2680, #31680, .T. ) ;
#4967=EDGE_CURVE ( 'NONE', #9213, #33021, #15040, .T. ) ;
#4999=DIRECTION ( 'NONE',  ( -0.2768435750659253847, -0.3568721902840677473, 0.8921882507333133150 ) ) ;
#5018=EDGE_CURVE ( 'NONE', #23812, #3754, #32809, .T. ) ;
#5038=ORIENTED_EDGE ( 'NONE', *, *, #9270, .F. ) ;
#5051=ORIENTED_EDGE ( 'NONE', *, *, #10574, .T. ) ;
#5080=VERTEX_POINT ( 'NONE', #30089 ) ;
#5108=AXIS2_PLACEMENT_3D ( 'NONE', #3903, #14855, #17821 ) ;
#5115=AXIS2_PLACEMENT_3D ( 'NONE', #6288, #20657, #9484 ) ;
#5121=FACE_OUTER_BOUND ( 'NONE', #34239, .T. ) ;
#5140=CARTESIAN_POINT ( 'NONE',  ( 70.19189222814998175, -62.26243369865490251, -38.10776559704283528 ) ) ;
#5159=VECTOR ( 'NONE', #17717, 1000.000000000000114 ) ;
#5165=CYLINDRICAL_SURFACE ( 'NONE', #6371, 3.000000000000001776 ) ;
#5167=EDGE_LOOP ( 'NONE', ( #4589, #3408, #5787, #27784, #30265, #1926 ) ) ;
#5191=ORIENTED_EDGE ( 'NONE', *, *, #495, .T. ) ;
#5199=ORIENTED_EDGE ( 'NONE', *, *, #39518, .T. ) ;
#5213=CARTESIAN_POINT ( 'NONE',  ( 70.19189222814998175, -54.47411573338475677, -34.99246555962335492 ) ) ;
#5218=AXIS2_PLACEMENT_3D ( 'NONE', #17388, #24232, #18276 ) ;
#5246=ORIENTED_EDGE ( 'NONE', *, *, #31182, .F. ) ;
#5262=EDGE_CURVE ( 'NONE', #17071, #38525, #36894, .T. ) ;
#5264=FACE_OUTER_BOUND ( 'NONE', #17363, .T. ) ;
#5273=EDGE_LOOP ( 'NONE', ( #19015, #20640, #32798, #23613, #3675 ) ) ;
#5280=ORIENTED_EDGE ( 'NONE', *, *, #3581, .T. ) ;
#5330=EDGE_CURVE ( 'NONE', #8760, #33236, #32592, .T. ) ;
#5365=ORIENTED_EDGE ( 'NONE', *, *, #25199, .T. ) ;
#5374=CARTESIAN_POINT ( 'NONE',  ( 70.19189222814998175, -52.97765562947117957, -34.39388673445118627 ) ) ;
#5384=CARTESIAN_POINT ( 'NONE',  ( 72.30589087944665039, -69.86246063582763099, -43.34095636271326413 ) ) ;
#5394=EDGE_CURVE ( 'NONE', #30461, #33992, #23480, .T. ) ;
#5396=DIRECTION ( 'NONE',  ( 0.2407039305251456596, -0.3604685577742790525, 0.9011792478113757054 ) ) ;
#5398=ORIENTED_EDGE ( 'NONE', *, *, #17508, .F. ) ;
#5403=DIRECTION ( 'NONE',  ( -0.000000000000000000, -0.9284778069183718952, -0.3713878862591649677 ) ) ;
#5428=ORIENTED_EDGE ( 'NONE', *, *, #29288, .F. ) ;
#5454=VECTOR ( 'NONE', #17973, 1000.000000000000227 ) ;
#5456=DIRECTION ( 'NONE',  ( 0.9609149988134837450, -0.1028163501681639419, 0.2570431154366518145 ) ) ;
#5508=CARTESIAN_POINT ( 'NONE',  ( 71.02242295334774269, -59.90284381096115851, -40.26874551563744831 ) ) ;
#5511=DIRECTION ( 'NONE',  ( -0.2768435750659241079, -0.3568721902840695792, 0.8921882507333129819 ) ) ;
#5529=CARTESIAN_POINT ( 'NONE',  ( 70.19189222814998175, -56.12358456014947450, -35.65224734057483857 ) ) ;
#5556=DIRECTION ( 'NONE',  ( -0.2768435750659241079, -0.3568721902840695792, 0.8921882507333129819 ) ) ;
#5569=ORIENTED_EDGE ( 'NONE', *, *, #37271, .T. ) ;
#5579=ORIENTED_EDGE ( 'NONE', *, *, #42493, .T. ) ;
#5590=CARTESIAN_POINT ( 'NONE',  ( 71.02242295334774269, -50.61806574177743556, -36.55486665304579930 ) ) ;
#5591=DIRECTION ( 'NONE',  ( -0.2407039305251456596, 0.3604685577742790525, -0.9011792478113757054 ) ) ;
#5602=DIRECTION ( 'NONE',  ( -0.000000000000000000, -0.9284778069183721172, -0.3713878862591650232 ) ) ;
#5615=ORIENTED_EDGE ( 'NONE', *, *, #38993, .F. ) ;
#5619=DIRECTION ( 'NONE',  ( -0.9609149988134837450, 0.1028163501681639419, -0.2570431154366518145 ) ) ;
#5625=ADVANCED_FACE ( 'NONE', ( #12993 ), #26889, .T. ) ;
#5656=ORIENTED_EDGE ( 'NONE', *, *, #3397, .F. ) ;
#5676=CARTESIAN_POINT ( 'NONE',  ( 69.36136150295220659, -101.1685209014307674, -50.56525720990386219 ) ) ;
#5681=DIRECTION ( 'NONE',  ( 0.9609149988134843001, -0.1028163501681632064, 0.2570431154366505933 ) ) ;
#5696=AXIS2_PLACEMENT_3D ( 'NONE', #25511, #36207, #36873 ) ;
#5700=CARTESIAN_POINT ( 'NONE',  ( 71.02242295334774269, -55.26045477636929348, -38.41180608434162025 ) ) ;
#5708=ORIENTED_EDGE ( 'NONE', *, *, #1349, .F. ) ;
#5748=ORIENTED_EDGE ( 'NONE', *, *, #7032, .T. ) ;
#5751=FACE_OUTER_BOUND ( 'NONE', #15622, .T. ) ;
#5782=ADVANCED_FACE ( 'NONE', ( #41926 ), #4839, .T. ) ;
#5784=EDGE_CURVE ( 'NONE', #11292, #6949, #1942, .T. ) ;
#5787=ORIENTED_EDGE ( 'NONE', *, *, #23104, .T. ) ;
#5798=DIRECTION ( 'NONE',  ( 0.9609149988134837450, -0.1028163501681639419, 0.2570431154366518145 ) ) ;
#5807=CARTESIAN_POINT ( 'NONE',  ( 73.07463722459043254, -51.06865355621575731, -32.73578466827673594 ) ) ;
#5840=CARTESIAN_POINT ( 'NONE',  ( 70.19189222814998175, -61.90193818873174791, -37.96356864969668266 ) ) ;
#5847=CARTESIAN_POINT ( 'NONE',  ( 67.84197459855160162, -53.65469605205331050, -35.39387355951068059 ) ) ;
#5892=AXIS2_PLACEMENT_3D ( 'NONE', #38720, #42616, #38952 ) ;
#5898=CARTESIAN_POINT ( 'NONE',  ( 73.07463722459043254, -57.56799820464436834, -35.33549987209089238 ) ) ;
#5911=DIRECTION ( 'NONE',  ( -0.000000000000000000, -0.9284778069183721172, -0.3713878862591650232 ) ) ;
#5912=DIRECTION ( 'NONE',  ( -0.000000000000000000, -0.9284778069183720062, -0.3713878862591650232 ) ) ;
#5935=DIRECTION ( 'NONE',  ( 0.000000000000000000, 0.9284778069183721172, 0.3713878862591650232 ) ) ;
#5938=AXIS2_PLACEMENT_3D ( 'NONE', #6094, #3129, #34131 ) ;
#5944=FACE_OUTER_BOUND ( 'NONE', #36058, .T. ) ;
#5955=VERTEX_POINT ( 'NONE', #11134 ) ;
#5956=EDGE_LOOP ( 'NONE', ( #41567, #44425, #31308, #25867 ) ) ;
#6016=CONICAL_SURFACE ( 'NONE', #8208, 2.541999999999999371, 1.047197551196596299 ) ;
#6017=CARTESIAN_POINT ( 'NONE',  ( 72.65915383727740107, -67.60605966022829705, -40.90420006524065144 ) ) ;
#6053=EDGE_CURVE ( 'NONE', #29144, #10520, #23820, .T. ) ;
#6079=CARTESIAN_POINT ( 'NONE',  ( 67.30914723170953096, -53.95817989580823593, -35.68060091436646530 ) ) ;
#6080=ADVANCED_FACE ( 'NONE', ( #26158 ), #32539, .T. ) ;
#6094=CARTESIAN_POINT ( 'NONE',  ( 70.19189222814998175, -54.83461124330791847, -35.13666250696951465 ) ) ;
#6097=EDGE_CURVE ( 'NONE', #44451, #30461, #1974, .T. ) ;
#6102=CIRCLE ( 'NONE', #280, 2.999999999999999556 ) ;
#6146=CARTESIAN_POINT ( 'NONE',  ( 65.38731723408255903, -64.53378536856919823, -40.50714483300358637 ) ) ;
#6157=EDGE_CURVE ( 'NONE', #19524, #35294, #4729, .T. ) ;
#6177=DIRECTION ( 'NONE',  ( -0.000000000000000000, -0.9284778069183718952, -0.3713878862591649677 ) ) ;
#6182=AXIS2_PLACEMENT_3D ( 'NONE', #38314, #6654, #41101 ) ;
#6184=DIRECTION ( 'NONE',  ( -0.7871354856660162103, -0.4483307682966942709, -0.4235767337848251879 ) ) ;
#6186=EDGE_LOOP ( 'NONE', ( #1401, #44303, #32862, #27899, #2709 ) ) ;
#6190=CIRCLE ( 'NONE', #16385, 2.445500000000004448 ) ;
#6204=CARTESIAN_POINT ( 'NONE',  ( 70.19189222814998175, -52.04917782255280656, -34.02249884819201498 ) ) ;
#6206=MANIFOLD_SOLID_BREP ( 'NONE', #17774 ) ;
#6232=ADVANCED_FACE ( 'NONE', ( #34116 ), #6538, .F. ) ;
#6239=ORIENTED_EDGE ( 'NONE', *, *, #2158, .T. ) ;
#6263=ORIENTED_EDGE ( 'NONE', *, *, #1622, .F. ) ;
#6288=CARTESIAN_POINT ( 'NONE',  ( 70.19189222814998175, -56.33107134722149567, -35.73524133214168330 ) ) ;
#6305=AXIS2_PLACEMENT_3D ( 'NONE', #27455, #37006, #5556 ) ;
#6308=DIRECTION ( 'NONE',  ( 0.9609149988134837450, -0.1028163501681639419, 0.2570431154366518145 ) ) ;
#6309=CARTESIAN_POINT ( 'NONE',  ( 72.54180985774836188, -62.51387108299115170, -37.47916665824249804 ) ) ;
#6310=FACE_OUTER_BOUND ( 'NONE', #20929, .T. ) ;
#6313=FACE_OUTER_BOUND ( 'NONE', #15783, .T. ) ;
#6371=AXIS2_PLACEMENT_3D ( 'NONE', #36394, #43260, #25707 ) ;
#6381=DIRECTION ( 'NONE',  ( -0.9609149988134837450, 0.1028163501681645109, -0.2570431154366520921 ) ) ;
#6398=ORIENTED_EDGE ( 'NONE', *, *, #11163, .T. ) ;
#6423=EDGE_CURVE ( 'NONE', #14508, #6975, #44186, .T. ) ;
#6432=CARTESIAN_POINT ( 'NONE',  ( 69.36136150295220659, -53.48028990332819177, -31.49013104333824131 ) ) ;
#6484=ORIENTED_EDGE ( 'NONE', *, *, #26163, .F. ) ;
#6499=LINE ( 'NONE', #27926, #40747 ) ;
#6510=CARTESIAN_POINT ( 'NONE',  ( 70.19189222814998175, -70.34019061884472990, -41.33884020749756871 ) ) ;
#6531=DIRECTION ( 'NONE',  ( -0.000000000000000000, -0.9284778069183721172, -0.3713878862591650232 ) ) ;
#6535=CYLINDRICAL_SURFACE ( 'NONE', #15506, 3.000000000000001776 ) ;
#6538=PLANE ( 'NONE',  #36177 ) ;
#6550=ORIENTED_EDGE ( 'NONE', *, *, #3028, .T. ) ;
#6551=DIRECTION ( 'NONE',  ( -0.2768435750659360983, -0.3568721902840809590, 0.8921882507333046552 ) ) ;
#6566=DIRECTION ( 'NONE',  ( 0.9609149988134837450, -0.1028163501681639419, 0.2570431154366518145 ) ) ;
#6588=CARTESIAN_POINT ( 'NONE',  ( 69.48536631248848039, -66.77523564985355620, -42.98127819198803934 ) ) ;
#6601=AXIS2_PLACEMENT_3D ( 'NONE', #38403, #28167, #27722 ) ;
#6611=EDGE_CURVE ( 'NONE', #13382, #44494, #32532, .T. ) ;
#6615=DIRECTION ( 'NONE',  ( -0.9609149988134837450, 0.1028163501681639419, -0.2570431154366518145 ) ) ;
#6632=EDGE_CURVE ( 'NONE', #40329, #39890, #38361, .T. ) ;
#6633=FACE_OUTER_BOUND ( 'NONE', #30966, .T. ) ;
#6651=ORIENTED_EDGE ( 'NONE', *, *, #1232, .T. ) ;
#6654=DIRECTION ( 'NONE',  ( -0.000000000000000000, -0.9284778069183721172, -0.3713878862591650232 ) ) ;
#6680=DIRECTION ( 'NONE',  ( -0.2768435750659241079, -0.3568721902840695792, 0.8921882507333129819 ) ) ;
#6685=DIRECTION ( 'NONE',  ( -0.000000000000000000, -0.9284778069183718952, -0.3713878862591649677 ) ) ;
#6705=DIRECTION ( 'NONE',  ( 0.000000000000000000, 0.9284778069183720062, 0.3713878862591650232 ) ) ;
#6725=DIRECTION ( 'NONE',  ( -0.2768435750659241079, -0.3568721902840695792, 0.8921882507333129819 ) ) ;
#6740=DIRECTION ( 'NONE',  ( -0.2768435750659243855, -0.3568721902840678029, 0.8921882507333135370 ) ) ;
#6759=CONICAL_SURFACE ( 'NONE', #11857, 2.999999999999999556, 0.9599310885968830309 ) ;
#6825=CARTESIAN_POINT ( 'NONE',  ( 69.48536631248848039, -66.77523564985355620, -42.98127819198803934 ) ) ;
#6830=AXIS2_PLACEMENT_3D ( 'NONE', #28636, #39112, #38877 ) ;
#6857=CARTESIAN_POINT ( 'NONE',  ( 69.36136150295220659, -101.1685209014307674, -50.56525720990386219 ) ) ;
#6872=ORIENTED_EDGE ( 'NONE', *, *, #9270, .T. ) ;
#6878=DIRECTION ( 'NONE',  ( 0.9609149988134843001, -0.1028163501681632064, 0.2570431154366505933 ) ) ;
#6886=ORIENTED_EDGE ( 'NONE', *, *, #11485, .F. ) ;
#6918=CARTESIAN_POINT ( 'NONE',  ( 69.36136150295220659, -101.1685209014307674, -50.56525720990386219 ) ) ;
#6920=ORIENTED_EDGE ( 'NONE', *, *, #5262, .F. ) ;
#6929=EDGE_LOOP ( 'NONE', ( #1898, #40656, #36045 ) ) ;
#6931=FACE_OUTER_BOUND ( 'NONE', #18754, .T. ) ;
#6935=DIRECTION ( 'NONE',  ( -0.2768435750659241079, -0.3568721902840686355, 0.8921882507333134260 ) ) ;
#6949=VERTEX_POINT ( 'NONE', #20409 ) ;
#6975=VERTEX_POINT ( 'NONE', #23148 ) ;
#6980=CARTESIAN_POINT ( 'NONE',  ( 70.19189222814998175, -61.69445140165969121, -37.88057465812982372 ) ) ;
#6989=DIRECTION ( 'NONE',  ( 0.9609149988134837450, -0.1028163501681639419, 0.2570431154366518145 ) ) ;
#6990=EDGE_CURVE ( 'NONE', #279, #34887, #32568, .T. ) ;
#7002=PLANE ( 'NONE',  #21211 ) ;
#7005=VECTOR ( 'NONE', #7514, 1000.000000000000114 ) ;
#7014=CARTESIAN_POINT ( 'NONE',  ( 70.19189222814998175, -55.19510675323109439, -35.28085945431567438 ) ) ;
#7018=ORIENTED_EDGE ( 'NONE', *, *, #36322, .T. ) ;
#7032=EDGE_CURVE ( 'NONE', #23460, #16741, #22469, .T. ) ;
#7033=AXIS2_PLACEMENT_3D ( 'NONE', #3822, #4275, #32087 ) ;
#7041=CARTESIAN_POINT ( 'NONE',  ( 70.19189222814998175, -50.76020450571126474, -33.50691401458669105 ) ) ;
#7075=CARTESIAN_POINT ( 'NONE',  ( 67.84197459855160162, -53.65469605205331050, -35.39387355951068059 ) ) ;
#7079=AXIS2_PLACEMENT_3D ( 'NONE', #41594, #6705, #21046 ) ;
#7094=CARTESIAN_POINT ( 'NONE',  ( 70.19189222814998175, -55.76308905022629858, -35.50805039322867884 ) ) ;
#7104=CARTESIAN_POINT ( 'NONE',  ( 71.02242295334774269, -99.02728775972636299, -55.91838671430374319 ) ) ;
#7111=ORIENTED_EDGE ( 'NONE', *, *, #16975, .F. ) ;
#7135=FACE_OUTER_BOUND ( 'NONE', #8986, .T. ) ;
#7171=CIRCLE ( 'NONE', #39918, 2.999999999999999556 ) ;
#7205=CARTESIAN_POINT ( 'NONE',  ( 70.19189222814998175, -66.47064387046886225, -39.79103499669764687 ) ) ;
#7220=CARTESIAN_POINT ( 'NONE',  ( 71.02242295334774269, -54.33197696945092758, -38.04041819808246316 ) ) ;
#7229=ORIENTED_EDGE ( 'NONE', *, *, #1232, .F. ) ;
#7246=LINE ( 'NONE', #6588, #16969 ) ;
#7289=CARTESIAN_POINT ( 'NONE',  ( 67.84197459855160162, -59.22556289356354142, -37.62220087706567284 ) ) ;
#7302=EDGE_LOOP ( 'NONE', ( #28989, #43092, #18629, #40157, #10590 ) ) ;
#7303=CONICAL_SURFACE ( 'NONE', #33484, 2.445500000000005336, 0.9599310885968757034 ) ;
#7354=CARTESIAN_POINT ( 'NONE',  ( 70.19189222814998175, -58.90901798090458641, -36.76641099935233825 ) ) ;
#7357=ORIENTED_EDGE ( 'NONE', *, *, #22236, .T. ) ;
#7378=ORIENTED_EDGE ( 'NONE', *, *, #44007, .F. ) ;
#7467=EDGE_LOOP ( 'NONE', ( #42947, #15317, #19668, #15546, #13937 ) ) ;
#7491=CARTESIAN_POINT ( 'NONE',  ( 70.19189222814998175, -60.76597359474132531, -37.50918677187066663 ) ) ;
#7514=DIRECTION ( 'NONE',  ( 0.7202110682883375858, 0.2576522076061144029, -0.6441361323747234469 ) ) ;
#7523=DIRECTION ( 'NONE',  ( 0.9609149988134843001, -0.1028163501681632064, 0.2570431154366505933 ) ) ;
#7527=AXIS2_PLACEMENT_3D ( 'NONE', #42365, #42814, #32529 ) ;
#7549=VECTOR ( 'NONE', #26072, 1000.000000000000227 ) ;
#7565=ORIENTED_EDGE ( 'NONE', *, *, #1349, .T. ) ;
#7597=DIRECTION ( 'NONE',  ( -0.9609149988134837450, 0.1028163501681639419, -0.2570431154366518145 ) ) ;
#7604=EDGE_CURVE ( 'NONE', #32855, #23460, #33415, .T. ) ;
#7625=CARTESIAN_POINT ( 'NONE',  ( 70.19189222814998175, -51.68868231262963775, -33.87830190084585524 ) ) ;
#7630=CARTESIAN_POINT ( 'NONE',  ( 72.54180985774836188, -61.58539327607277869, -37.10777877198333385 ) ) ;
#7655=EDGE_CURVE ( 'NONE', #37519, #10810, #2118, .T. ) ;
#7690=CARTESIAN_POINT ( 'NONE',  ( 67.37136766119182596, -70.31694239570130378, -42.20474206142759499 ) ) ;
#7691=CARTESIAN_POINT ( 'NONE',  ( 71.02242295334774269, -49.63644658180010083, -36.16222241080433264 ) ) ;
#7692=ORIENTED_EDGE ( 'NONE', *, *, #1112, .T. ) ;
#7702=DIRECTION ( 'NONE',  ( -0.000000000000000000, -0.9284778069183721172, -0.3713878862591650232 ) ) ;
#7705=DIRECTION ( 'NONE',  ( 0.2768435750659235528, 0.3568721902840663041, -0.8921882507333145362 ) ) ;
#7706=VECTOR ( 'NONE', #40235, 1000.000000000000114 ) ;
#7714=CARTESIAN_POINT ( 'NONE',  ( 69.36136150295220659, -101.1685209014307674, -50.56525720990386219 ) ) ;
#7722=DIRECTION ( 'NONE',  ( 0.7871354856660167654, -0.6167752151498625546, -0.002461946824136807422 ) ) ;
#7741=DIRECTION ( 'NONE',  ( -0.2768435750659241079, -0.3568721902840695792, 0.8921882507333129819 ) ) ;
#7746=ADVANCED_FACE ( 'NONE', ( #26068 ), #16033, .F. ) ;
#7751=PRODUCT_DEFINITION_SHAPE ( 'NONE', 'NONE',  #9359 ) ;
#7753=CARTESIAN_POINT ( 'NONE',  ( 70.19189222814998175, -57.62004466406304459, -36.25082616574700722 ) ) ;
#7777=ORIENTED_EDGE ( 'NONE', *, *, #2248, .T. ) ;
#7786=ORIENTED_EDGE ( 'NONE', *, *, #38125, .F. ) ;
#7793=DIRECTION ( 'NONE',  ( -0.000000000000000000, -0.9284778069183721172, -0.3713878862591650232 ) ) ;
#7809=CARTESIAN_POINT ( 'NONE',  ( 70.19189222814998175, -60.04498257489500190, -37.22079287717834717 ) ) ;
#7862=EDGE_CURVE ( 'NONE', #11704, #12164, #42204, .T. ) ;
#7871=EDGE_CURVE ( 'NONE', #38683, #14232, #23258, .T. ) ;
#7884=DIRECTION ( 'NONE',  ( -0.2768435750659241079, -0.3568721902840695792, 0.8921882507333129819 ) ) ;
#7887=AXIS2_PLACEMENT_3D ( 'NONE', #12742, #40558, #9318 ) ;
#7930=DIRECTION ( 'NONE',  ( -0.9609149988134837450, 0.1028163501681639419, -0.2570431154366518145 ) ) ;
#7933=CARTESIAN_POINT ( 'NONE',  ( 68.80767435282035649, -72.12455157026508346, -36.87789895383100003 ) ) ;
#7948=DIRECTION ( 'NONE',  ( -0.000000000000000000, -0.9284778069183721172, -0.3713878862591650232 ) ) ;
#7981=EDGE_LOOP ( 'NONE', ( #4086, #3955, #44211, #39839, #37228 ) ) ;
#7985=CARTESIAN_POINT ( 'NONE',  ( 70.19189222814998175, -100.0979043305785581, -53.24182196210380624 ) ) ;
#7988=CARTESIAN_POINT ( 'NONE',  ( 72.30589087944665039, -67.07702721507251908, -42.22679270393576445 ) ) ;
#8008=DIRECTION ( 'NONE',  ( -0.000000000000000000, -0.9284778069183720062, -0.3713878862591650232 ) ) ;
#8026=ORIENTED_EDGE ( 'NONE', *, *, #25222, .F. ) ;
#8028=CIRCLE ( 'NONE', #24057, 2.999999999999999556 ) ;
#8059=EDGE_CURVE ( 'NONE', #36514, #37519, #6499, .T. ) ;
#8102=DIRECTION ( 'NONE',  ( -0.9609149988134836340, 0.1028163501681645525, -0.2570431154366521476 ) ) ;
#8134=CARTESIAN_POINT ( 'NONE',  ( 70.19189222814998175, -56.12358456014947450, -35.65224734057483857 ) ) ;
#8155=ORIENTED_EDGE ( 'NONE', *, *, #2158, .F. ) ;
#8161=CARTESIAN_POINT ( 'NONE',  ( 70.19189222814998175, -100.0979043305785581, -53.24182196210380624 ) ) ;
#8168=DIRECTION ( 'NONE',  ( -0.000000000000000000, -0.9284778069183718952, -0.3713878862591649677 ) ) ;
#8181=EDGE_CURVE ( 'NONE', #20803, #24054, #11263, .T. ) ;
#8182=LINE ( 'NONE', #22532, #16758 ) ;
#8191=VECTOR ( 'NONE', #45119, 1000.000000000000227 ) ;
#8193=CARTESIAN_POINT ( 'NONE',  ( 73.07463722459043254, -59.42495381848112856, -36.07827564460922787 ) ) ;
#8208=AXIS2_PLACEMENT_3D ( 'NONE', #30799, #20985, #38081 ) ;
#8209=FACE_OUTER_BOUND ( 'NONE', #6929, .T. ) ;
#8220=AXIS2_PLACEMENT_3D ( 'NONE', #8548, #22449, #32915 ) ;
#8251=UNCERTAINTY_MEASURE_WITH_UNIT (LENGTH_MEASURE( 1.000000000000000082E-05 ), #25752, 'distance_accuracy_value', 'NONE');
#8259=ORIENTED_EDGE ( 'NONE', *, *, #14994, .F. ) ;
#8269=EDGE_CURVE ( 'NONE', #18421, #43489, #24709, .T. ) ;
#8273=CARTESIAN_POINT ( 'NONE',  ( 70.19189222814998175, -56.12358456014947450, -35.65224734057483857 ) ) ;
#8282=ORIENTED_EDGE ( 'NONE', *, *, #44579, .T. ) ;
#8287=CARTESIAN_POINT ( 'NONE',  ( 67.30914723170953096, -52.10122428197148992, -34.93782514184813692 ) ) ;
#8341=VERTEX_POINT ( 'NONE', #30552 ) ;
#8353=CARTESIAN_POINT ( 'NONE',  ( 73.07463722459043254, -55.71104259080762233, -34.59272409957256400 ) ) ;
#8362=CARTESIAN_POINT ( 'NONE',  ( 67.84197459855160162, -61.08251850740028033, -38.36497664958400122 ) ) ;
#8371=CIRCLE ( 'NONE', #42611, 2.999999999999999556 ) ;
#8374=FACE_OUTER_BOUND ( 'NONE', #9618, .T. ) ;
#8375=CARTESIAN_POINT ( 'NONE',  ( 70.19189222814998175, -52.61716011954800365, -34.24968978710501943 ) ) ;
#8383=ADVANCED_FACE ( 'NONE', ( #23503 ), #26089, .T. ) ;
#8386=CYLINDRICAL_SURFACE ( 'NONE', #15683, 3.000000000000001776 ) ;
#8387=EDGE_CURVE ( 'NONE', #23245, #19524, #12264, .T. ) ;
#8414=CARTESIAN_POINT ( 'NONE',  ( 67.84197459855160162, -52.72621824513493038, -35.02248567325151640 ) ) ;
#8416=ORIENTED_EDGE ( 'NONE', *, *, #40344, .F. ) ;
#8420=CARTESIAN_POINT ( 'NONE',  ( 67.30914723170953096, -54.16566668288025710, -35.76359490593331003 ) ) ;
#8421=CARTESIAN_POINT ( 'NONE',  ( 73.01241679510815175, -70.92052552613920113, -40.69577108532303811 ) ) ;
#8442=FACE_OUTER_BOUND ( 'NONE', #42845, .T. ) ;
#8456=CARTESIAN_POINT ( 'NONE',  ( 67.84197459855160162, -56.44012947280842241, -36.50803721828817316 ) ) ;
#8464=CARTESIAN_POINT ( 'NONE',  ( 70.19189222814998175, -55.40259354030312267, -35.36385344588251911 ) ) ;
#8482=DIRECTION ( 'NONE',  ( -0.000000000000000000, -0.9284778069183721172, -0.3713878862591650232 ) ) ;
#8514=ORIENTED_EDGE ( 'NONE', *, *, #8613, .T. ) ;
#8516=DIRECTION ( 'NONE',  ( -0.000000000000000000, -0.9284778069183718952, -0.3713878862591649677 ) ) ;
#8536=AXIS2_PLACEMENT_3D ( 'NONE', #4000, #591, #38882 ) ;
#8547=DIRECTION ( 'NONE',  ( 0.9609149988134843001, -0.1028163501681632064, 0.2570431154366505933 ) ) ;
#8548=CARTESIAN_POINT ( 'NONE',  ( 70.19189222814998175, -51.68868231262963775, -33.87830190084585524 ) ) ;
#8556=ORIENTED_EDGE ( 'NONE', *, *, #11389, .T. ) ;
#8567=ORIENTED_EDGE ( 'NONE', *, *, #587, .T. ) ;
#8582=EDGE_CURVE ( 'NONE', #34725, #29032, #7171, .T. ) ;
#8588=EDGE_CURVE ( 'NONE', #34274, #33082, #4331, .T. ) ;
#8603=CARTESIAN_POINT ( 'NONE',  ( 72.54180985774836188, -60.65691546915440568, -36.73639088572416966 ) ) ;
#8611=DIRECTION ( 'NONE',  ( -0.2768435750659241079, -0.3568721902840695792, 0.8921882507333129819 ) ) ;
#8613=EDGE_CURVE ( 'NONE', #5955, #24054, #2777, .T. ) ;
#8617=ADVANCED_FACE ( 'NONE', ( #25288 ), #12363, .T. ) ;
#8659=DIRECTION ( 'NONE',  ( 0.9609149988134837450, -0.1028163501681639419, 0.2570431154366518145 ) ) ;
#8664=CARTESIAN_POINT ( 'NONE',  ( 70.19189222814998175, -59.83749578782295941, -37.13779888561150244 ) ) ;
#8665=CIRCLE ( 'NONE', #29794, 2.445500000000005336 ) ;
#8666=DIRECTION ( 'NONE',  ( -0.000000000000000000, -0.9284778069183720062, -0.3713878862591650232 ) ) ;
#8682=ORIENTED_EDGE ( 'NONE', *, *, #7862, .T. ) ;
#8691=CARTESIAN_POINT ( 'NONE',  ( 73.07463722459043254, -60.35343162539949446, -36.44966353086839206 ) ) ;
#8699=ORIENTED_EDGE ( 'NONE', *, *, #10836, .F. ) ;
#8701=CIRCLE ( 'NONE', #10894, 2.999999999999999556 ) ;
#8729=CARTESIAN_POINT ( 'NONE',  ( 70.19189222814998175, -59.83749578782295941, -37.13779888561150244 ) ) ;
#8743=CIRCLE ( 'NONE', #40052, 2.999999999999999556 ) ;
#8760=VERTEX_POINT ( 'NONE', #9082 ) ;
#8777=ORIENTED_EDGE ( 'NONE', *, *, #42324, .F. ) ;
#8796=LINE ( 'NONE', #43007, #23813 ) ;
#8807=CARTESIAN_POINT ( 'NONE',  ( 71.02242295334774269, -99.02728775972636299, -55.91838671430374319 ) ) ;
#8808=EDGE_LOOP ( 'NONE', ( #3050, #23553, #36226, #44641, #43126 ) ) ;
#8812=AXIS2_PLACEMENT_3D ( 'NONE', #20983, #13919, #21202 ) ;
#8815=VECTOR ( 'NONE', #8913, 1000.000000000000114 ) ;
#8858=DIRECTION ( 'NONE',  ( -0.2768435750659239414, -0.3568721902840664151, 0.8921882507333142032 ) ) ;
#8868=FACE_OUTER_BOUND ( 'NONE', #38724, .T. ) ;
#8870=EDGE_CURVE ( 'NONE', #2680, #5955, #10796, .T. ) ;
#8876=DIRECTION ( 'NONE',  ( -0.000000000000000000, -0.9284778069183721172, -0.3713878862591650232 ) ) ;
#8886=DIRECTION ( 'NONE',  ( 0.9609149988134837450, -0.1028163501681639419, 0.2570431154366518145 ) ) ;
#8913=DIRECTION ( 'NONE',  ( -0.9609149988134834119, 0.1028163501681648995, -0.2570431154366529802 ) ) ;
#8940=ADVANCED_FACE ( 'NONE', ( #32346 ), #11609, .T. ) ;
#8943=VERTEX_POINT ( 'NONE', #39423 ) ;
#8951=CYLINDRICAL_SURFACE ( 'NONE', #28449, 3.000000000000001776 ) ;
#8960=CIRCLE ( 'NONE', #31534, 2.999999999999999556 ) ;
#8961=DIRECTION ( 'NONE',  ( -0.000000000000000000, -0.9284778069183718952, -0.3713878862591649677 ) ) ;
#8963=CARTESIAN_POINT ( 'NONE',  ( 70.86891319097370001, -49.31949126737637812, -35.46156944284200563 ) ) ;
#8972=CARTESIAN_POINT ( 'NONE',  ( 73.07463722459043254, -59.21746703140907897, -35.99528165304237604 ) ) ;
#8986=EDGE_LOOP ( 'NONE', ( #32423, #41248, #12929, #34150, #42729 ) ) ;
#8995=TOROIDAL_SURFACE ( 'NONE', #41777, 4.700000000000000178, 0.2999999999999999889 ) ;
#9007=DIRECTION ( 'NONE',  ( -0.7871354856660202071, 0.6167752151498580027, 0.002461946824133919541 ) ) ;
#9017=DIRECTION ( 'NONE',  ( 0.9609149988134837450, -0.1028163501681639419, 0.2570431154366518145 ) ) ;
#9056=CARTESIAN_POINT ( 'NONE',  ( 69.36136150295220659, -52.75929888348183994, -31.20173714864591830 ) ) ;
#9082=CARTESIAN_POINT ( 'NONE',  ( 69.36136150295220659, -58.12267893792004259, -33.34707047463405871 ) ) ;
#9084=CARTESIAN_POINT ( 'NONE',  ( 72.30589087944665039, -67.07702721507251908, -42.22679270393576445 ) ) ;
#9098=LINE ( 'NONE', #33698, #35131 ) ;
#9103=DIRECTION ( 'NONE',  ( -0.9609149988134837450, 0.1028163501681639419, -0.2570431154366518145 ) ) ;
#9114=DIRECTION ( 'NONE',  ( 0.000000000000000000, 0.9284778069183720062, 0.3713878862591650232 ) ) ;
#9118=EDGE_CURVE ( 'NONE', #2964, #44682, #14436, .T. ) ;
#9152=LINE ( 'NONE', #40618, #9650 ) ;
#9162=ORIENTED_EDGE ( 'NONE', *, *, #27531, .T. ) ;
#9170=AXIS2_PLACEMENT_3D ( 'NONE', #37507, #2395, #16324 ) ;
#9185=ADVANCED_FACE ( 'NONE', ( #29835 ), #19573, .T. ) ;
#9209=LINE ( 'NONE', #27829, #11029 ) ;
#9213=VERTEX_POINT ( 'NONE', #8414 ) ;
#9220=EDGE_CURVE ( 'NONE', #34283, #42441, #45046, .T. ) ;
#9222=AXIS2_PLACEMENT_3D ( 'NONE', #38744, #4083, #7741 ) ;
#9236=EDGE_LOOP ( 'NONE', ( #16536, #8514, #19385, #43081, #20711, #39419 ) ) ;
#9251=VECTOR ( 'NONE', #3394, 1000.000000000000227 ) ;
#9266=ORIENTED_EDGE ( 'NONE', *, *, #41493, .T. ) ;
#9270=EDGE_CURVE ( 'NONE', #9298, #38344, #25380, .T. ) ;
#9272=CIRCLE ( 'NONE', #28922, 2.999999999999999556 ) ;
#9282=EDGE_LOOP ( 'NONE', ( #39307, #16680, #11885, #11488, #22212 ) ) ;
#9294=VECTOR ( 'NONE', #22862, 1000.000000000000000 ) ;
#9298=VERTEX_POINT ( 'NONE', #44432 ) ;
#9318=DIRECTION ( 'NONE',  ( 0.9609149988134843001, -0.1028163501681632064, 0.2570431154366505933 ) ) ;
#9320=EDGE_LOOP ( 'NONE', ( #24900, #23436, #34370, #9353, #45004, #33871 ) ) ;
#9340=CARTESIAN_POINT ( 'NONE',  ( 67.30914723170953096, -62.31448015807357166, -39.02309189069894302 ) ) ;
#9353=ORIENTED_EDGE ( 'NONE', *, *, #12252, .T. ) ;
#9359=PRODUCT_DEFINITION ( 'UNKNOWN', '', #28600, #4596 ) ;
#9369=ORIENTED_EDGE ( 'NONE', *, *, #22760, .T. ) ;
#9388=ORIENTED_EDGE ( 'NONE', *, *, #33755, .T. ) ;
#9399=FACE_OUTER_BOUND ( 'NONE', #21695, .T. ) ;
#9420=ORIENTED_EDGE ( 'NONE', *, *, #40344, .T. ) ;
#9431=VERTEX_POINT ( 'NONE', #16384 ) ;
#9437=ORIENTED_EDGE ( 'NONE', *, *, #38993, .T. ) ;
#9438=FACE_OUTER_BOUND ( 'NONE', #32639, .T. ) ;
#9459=DIRECTION ( 'NONE',  ( 0.9609149988134837450, -0.1028163501681639419, 0.2570431154366518145 ) ) ;
#9469=CONICAL_SURFACE ( 'NONE', #731, 2.445500000000004448, 0.9599310885968757034 ) ;
#9475=FACE_OUTER_BOUND ( 'NONE', #24147, .T. ) ;
#9484=DIRECTION ( 'NONE',  ( 0.9609149988134837450, -0.1028163501681639419, 0.2570431154366518145 ) ) ;
#9495=ORIENTED_EDGE ( 'NONE', *, *, #14542, .T. ) ;
#9520=EDGE_CURVE ( 'NONE', #22284, #43627, #18853, .T. ) ;
#9537=DIRECTION ( 'NONE',  ( 0.2768435750659235528, 0.3568721902840663041, -0.8921882507333145362 ) ) ;
#9545=ORIENTED_EDGE ( 'NONE', *, *, #25043, .F. ) ;
#9567=CARTESIAN_POINT ( 'NONE',  ( 71.02242295334774269, -99.02728775972636299, -55.91838671430374319 ) ) ;
#9618=EDGE_LOOP ( 'NONE', ( #44476, #32317, #14413, #27307, #14116, #1101 ) ) ;
#9620=VECTOR ( 'NONE', #27895, 1000.000000000000114 ) ;
#9650=VECTOR ( 'NONE', #23284, 1000.000000000000227 ) ;
#9656=CIRCLE ( 'NONE', #169, 2.445500000000005336 ) ;
#9672=EDGE_CURVE ( 'NONE', #31689, #3470, #8665, .T. ) ;
#9679=CONICAL_SURFACE ( 'NONE', #22746, 2.999999999999999556, 0.9599310885968830309 ) ;
#9682=CIRCLE ( 'NONE', #26408, 2.999999999999999556 ) ;
#9683=CARTESIAN_POINT ( 'NONE',  ( 70.19189222814998175, -56.69156685714467159, -35.87943827948784303 ) ) ;
#9699=VERTEX_POINT ( 'NONE', #14306 ) ;
#9754=ORIENTED_EDGE ( 'NONE', *, *, #10899, .T. ) ;
#9778=VERTEX_POINT ( 'NONE', #36164 ) ;
#9782=( NAMED_UNIT ( * ) PLANE_ANGLE_UNIT ( ) SI_UNIT ( $, .RADIAN. ) );
#9800=CARTESIAN_POINT ( 'NONE',  ( 71.02242295334774269, -99.02728775972636299, -55.91838671430374319 ) ) ;
#9828=ADVANCED_FACE ( 'NONE', ( #39823 ), #16696, .T. ) ;
#9852=AXIS2_PLACEMENT_3D ( 'NONE', #27473, #27697, #44804 ) ;
#9863=CARTESIAN_POINT ( 'NONE',  ( 71.09163384711422395, -63.65591304925720095, -42.02869409913880361 ) ) ;
#9897=CARTESIAN_POINT ( 'NONE',  ( 70.19189222814998175, -52.04917782255280656, -34.02249884819201498 ) ) ;
#9918=DIRECTION ( 'NONE',  ( 0.9609149988134843001, -0.1028163501681632064, 0.2570431154366505933 ) ) ;
#9946=CARTESIAN_POINT ( 'NONE',  ( 69.36136150295220659, -56.26572332408330368, -32.60429470211573033 ) ) ;
#9958=ORIENTED_EDGE ( 'NONE', *, *, #17407, .F. ) ;
#9963=DIRECTION ( 'NONE',  ( 0.2768435750659263284, 0.3568721902840676363, -0.8921882507333129819 ) ) ;
#9983=ORIENTED_EDGE ( 'NONE', *, *, #14309, .F. ) ;
#10017=EDGE_CURVE ( 'NONE', #22169, #40557, #28361, .T. ) ;
#10029=AXIS2_PLACEMENT_3D ( 'NONE', #33824, #2594, #8547 ) ;
#10032=LINE ( 'NONE', #9567, #35277 ) ;
#10034=DIRECTION ( 'NONE',  ( 0.9609149988134843001, -0.1028163501681632064, 0.2570431154366505933 ) ) ;
#10044=EDGE_CURVE ( 'NONE', #44794, #9699, #8701, .T. ) ;
#10077=ORIENTED_EDGE ( 'NONE', *, *, #20144, .F. ) ;
#10089=CARTESIAN_POINT ( 'NONE',  ( 73.07463722459043254, -62.21038723923624048, -37.19243930338672754 ) ) ;
#10093=CARTESIAN_POINT ( 'NONE',  ( 71.49305703095983233, -68.94143466658512409, -45.64354135182188799 ) ) ;
#10120=LINE ( 'NONE', #40670, #12172 ) ;
#10137=LINE ( 'NONE', #10578, #20238 ) ;
#10140=CARTESIAN_POINT ( 'NONE',  ( 70.19189222814998175, -51.68868231262963775, -33.87830190084585524 ) ) ;
#10144=CARTESIAN_POINT ( 'NONE',  ( 67.84197459855160162, -50.86926263129819148, -34.27970990073318802 ) ) ;
#10145=ORIENTED_EDGE ( 'NONE', *, *, #10574, .F. ) ;
#10149=FACE_OUTER_BOUND ( 'NONE', #9320, .T. ) ;
#10157=VECTOR ( 'NONE', #18097, 1000.000000000000000 ) ;
#10185=AXIS2_PLACEMENT_3D ( 'NONE', #26704, #29897, #33981 ) ;
#10194=CIRCLE ( 'NONE', #22570, 2.999999999999999556 ) ;
#10215=AXIS2_PLACEMENT_3D ( 'NONE', #25061, #429, #14346 ) ;
#10246=CIRCLE ( 'NONE', #17521, 2.445500000000004448 ) ;
#10253=CONICAL_SURFACE ( 'NONE', #12429, 2.445500000000004448, 0.9599310885968757034 ) ;
#10287=VERTEX_POINT ( 'NONE', #9946 ) ;
#10304=ORIENTED_EDGE ( 'NONE', *, *, #14423, .T. ) ;
#10311=DIRECTION ( 'NONE',  ( 0.9609149988134838560, -0.1028163501681645386, 0.2570431154366520921 ) ) ;
#10329=DIRECTION ( 'NONE',  ( -0.000000000000000000, -0.9284778069183721172, -0.3713878862591650232 ) ) ;
#10334=CARTESIAN_POINT ( 'NONE',  ( 70.19189222814998175, -58.54852247098141049, -36.62221405200617141 ) ) ;
#10336=VERTEX_POINT ( 'NONE', #38401 ) ;
#10337=DIRECTION ( 'NONE',  ( 0.9609149988134843001, -0.1028163501681632064, 0.2570431154366505933 ) ) ;
#10350=DIRECTION ( 'NONE',  ( -0.000000000000000000, -0.9284778069183721172, -0.3713878862591650232 ) ) ;
#10361=DIRECTION ( 'NONE',  ( 0.9609149988134843001, -0.1028163501681632064, 0.2570431154366505933 ) ) ;
#10412=CARTESIAN_POINT ( 'NONE',  ( 69.36136150295220659, -59.05115674483842270, -33.71845836089322290 ) ) ;
#10432=CIRCLE ( 'NONE', #34428, 3.000000000000001776 ) ;
#10437=AXIS2_PLACEMENT_3D ( 'NONE', #30174, #24836, #31444 ) ;
#10458=ADVANCED_FACE ( 'NONE', ( #12579 ), #26249, .T. ) ;
#10469=VECTOR ( 'NONE', #6177, 1000.000000000000227 ) ;
#10488=DIRECTION ( 'NONE',  ( -0.000000000000000000, -0.9284778069183721172, -0.3713878862591650232 ) ) ;
#10519=ORIENTED_EDGE ( 'NONE', *, *, #12380, .T. ) ;
#10520=VERTEX_POINT ( 'NONE', #28174 ) ;
#10542=ORIENTED_EDGE ( 'NONE', *, *, #2301, .T. ) ;
#10555=CONICAL_SURFACE ( 'NONE', #40394, 2.999999999999999556, 0.9599310885968830309 ) ;
#10556=ORIENTED_EDGE ( 'NONE', *, *, #2559, .T. ) ;
#10574=EDGE_CURVE ( 'NONE', #14508, #4821, #21544, .T. ) ;
#10578=CARTESIAN_POINT ( 'NONE',  ( 70.89841814381148311, -68.89136543047671069, -37.69090763720760151 ) ) ;
#10590=ORIENTED_EDGE ( 'NONE', *, *, #23388, .F. ) ;
#10615=FACE_OUTER_BOUND ( 'NONE', #33302, .T. ) ;
#10616=ADVANCED_FACE ( 'NONE', ( #16251 ), #24710, .T. ) ;
#10634=AXIS2_PLACEMENT_3D ( 'NONE', #14023, #24071, #37739 ) ;
#10657=ADVANCED_FACE ( 'NONE', ( #9399 ), #25475, .T. ) ;
#10665=DIRECTION ( 'NONE',  ( 0.9609149988134837450, -0.1028163501681639419, 0.2570431154366518145 ) ) ;
#10675=VECTOR ( 'NONE', #18338, 1000.000000000000114 ) ;
#10690=DIRECTION ( 'NONE',  ( -0.9609149988134837450, 0.1028163501681639419, -0.2570431154366518145 ) ) ;
#10703=ORIENTED_EDGE ( 'NONE', *, *, #34780, .F. ) ;
#10707=CARTESIAN_POINT ( 'NONE',  ( 73.07463722459043254, -53.64660018989884804, -33.76695433548739089 ) ) ;
#10721=ORIENTED_EDGE ( 'NONE', *, *, #15840, .F. ) ;
#10727=DIRECTION ( 'NONE',  ( 1.000000000000000000, 0.000000000000000000, 0.000000000000000000 ) ) ;
#10764=AXIS2_PLACEMENT_3D ( 'NONE', #8729, #21967, #15128 ) ;
#10773=DIRECTION ( 'NONE',  ( -0.2768435750659253847, -0.3568721902840677473, 0.8921882507333133150 ) ) ;
#10796=CIRCLE ( 'NONE', #5696, 2.999999999999999556 ) ;
#10802=CARTESIAN_POINT ( 'NONE',  ( 67.37136766119182596, -67.53150897494617766, -41.09057840265009531 ) ) ;
#10805=SHAPE_REPRESENTATION ( 'Clamp Bolt', ( #12375 ), #32596 ) ;
#10810=VERTEX_POINT ( 'NONE', #20574 ) ;
#10836=EDGE_CURVE ( 'NONE', #38525, #37456, #11632, .T. ) ;
#10866=CARTESIAN_POINT ( 'NONE',  ( 70.19189222814998175, -67.83330054016514055, -40.33609291459782753 ) ) ;
#10871=ORIENTED_EDGE ( 'NONE', *, *, #20893, .F. ) ;
#10894=AXIS2_PLACEMENT_3D ( 'NONE', #31945, #29432, #18277 ) ;
#10899=EDGE_CURVE ( 'NONE', #8943, #38525, #14391, .T. ) ;
#10934=DIRECTION ( 'NONE',  ( -0.7871354856660202071, 0.6167752151498580027, 0.002461946824133919541 ) ) ;
#10945=DIRECTION ( 'NONE',  ( -0.000000000000000000, -0.9284778069183721172, -0.3713878862591650232 ) ) ;
#10951=ORIENTED_EDGE ( 'NONE', *, *, #17533, .T. ) ;
#10953=CARTESIAN_POINT ( 'NONE',  ( 73.07463722459043254, -51.99713136313413031, -33.10717255453590013 ) ) ;
#10962=CIRCLE ( 'NONE', #37911, 2.999999999999999556 ) ;
#10984=VECTOR ( 'NONE', #2571, 999.9999999999998863 ) ;
#11005=AXIS2_PLACEMENT_3D ( 'NONE', #384, #28214, #4019 ) ;
#11009=ORIENTED_EDGE ( 'NONE', *, *, #5018, .T. ) ;
#11029=VECTOR ( 'NONE', #16048, 1000.000000000000000 ) ;
#11030=CARTESIAN_POINT ( 'NONE',  ( 69.36136150295220659, -51.83082107656346693, -30.83034926238675411 ) ) ;
#11046=CARTESIAN_POINT ( 'NONE',  ( 69.48536631248848039, -69.56066907060868232, -44.09544185076553191 ) ) ;
#11049=CARTESIAN_POINT ( 'NONE',  ( 70.19189222814998175, -54.26662894631272849, -34.90947156805651019 ) ) ;
#11058=DIRECTION ( 'NONE',  ( -0.000000000000000000, -0.9284778069183721172, -0.3713878862591650232 ) ) ;
#11116=CONICAL_SURFACE ( 'NONE', #43203, 2.999999999999999556, 0.9599310885968830309 ) ;
#11134=CARTESIAN_POINT ( 'NONE',  ( 71.02242295334774269, -58.76687921697075723, -39.81436363781143228 ) ) ;
#11142=ADVANCED_FACE ( 'NONE', ( #32167 ), #32762, .T. ) ;
#11148=DIRECTION ( 'NONE',  ( 0.000000000000000000, 0.9284778069183720062, 0.3713878862591650232 ) ) ;
#11156=LINE ( 'NONE', #44930, #38589 ) ;
#11163=EDGE_CURVE ( 'NONE', #33002, #19823, #35670, .T. ) ;
#11166=ORIENTED_EDGE ( 'NONE', *, *, #26228, .T. ) ;
#11177=CARTESIAN_POINT ( 'NONE',  ( 67.37136766119182596, -67.53150897494617766, -41.09057840265009531 ) ) ;
#11198=CARTESIAN_POINT ( 'NONE',  ( 70.19189222814998175, -57.62004466406304459, -36.25082616574700722 ) ) ;
#11240=AXIS2_PLACEMENT_3D ( 'NONE', #44294, #41102, #20345 ) ;
#11250=CARTESIAN_POINT ( 'NONE',  ( 67.30914723170953096, -60.45752454423683275, -38.28031611818062174 ) ) ;
#11263=LINE ( 'NONE', #4180, #10157 ) ;
#11292=VERTEX_POINT ( 'NONE', #12335 ) ;
#11305=DIRECTION ( 'NONE',  ( -0.000000000000000000, -0.9284778069183721172, -0.3713878862591650232 ) ) ;
#11315=ORIENTED_EDGE ( 'NONE', *, *, #1112, .F. ) ;
#11338=VECTOR ( 'NONE', #28335, 1000.000000000000227 ) ;
#11349=ORIENTED_EDGE ( 'NONE', *, *, #40755, .F. ) ;
#11359=ADVANCED_FACE ( 'NONE', ( #26235 ), #25499, .T. ) ;
#11376=ORIENTED_EDGE ( 'NONE', *, *, #33178, .T. ) ;
#11389=EDGE_CURVE ( 'NONE', #42441, #34283, #29135, .T. ) ;
#11390=AXIS2_PLACEMENT_3D ( 'NONE', #37774, #12947, #38002 ) ;
#11405=AXIS2_PLACEMENT_3D ( 'NONE', #1418, #15117, #12376 ) ;
#11420=ADVANCED_FACE ( 'NONE', ( #44706 ), #26213, .T. ) ;
#11435=ORIENTED_EDGE ( 'NONE', *, *, #23104, .F. ) ;
#11442=ORIENTED_EDGE ( 'NONE', *, *, #30988, .T. ) ;
#11447=LINE ( 'NONE', #16156, #34942 ) ;
#11467=ORIENTED_EDGE ( 'NONE', *, *, #7032, .F. ) ;
#11485=EDGE_CURVE ( 'NONE', #31092, #13251, #11156, .T. ) ;
#11488=ORIENTED_EDGE ( 'NONE', *, *, #25570, .F. ) ;
#11490=LINE ( 'NONE', #39066, #28432 ) ;
#11491=CARTESIAN_POINT ( 'NONE',  ( 70.19189222814998175, -50.19222220871606766, -33.27972307567368659 ) ) ;
#11528=DIRECTION ( 'NONE',  ( -0.000000000000000000, -0.9284778069183721172, -0.3713878862591650232 ) ) ;
#11556=ADVANCED_FACE ( 'NONE', ( #17330 ), #38065, .T. ) ;
#11565=EDGE_LOOP ( 'NONE', ( #12650, #23778, #10556, #37976, #28797, #26274 ) ) ;
#11566=DIRECTION ( 'NONE',  ( -0.2768435750659243300, -0.3568721902840674698, 0.8921882507333136481 ) ) ;
#11595=DIRECTION ( 'NONE',  ( 0.9609149988134843001, -0.1028163501681632064, 0.2570431154366505933 ) ) ;
#11609=PLANE ( 'NONE',  #36258 ) ;
#11632=CIRCLE ( 'NONE', #37097, 2.999999999999999556 ) ;
#11637=EDGE_CURVE ( 'NONE', #28070, #26037, #18200, .T. ) ;
#11649=EDGE_CURVE ( 'NONE', #33082, #9431, #42239, .T. ) ;
#11660=DIRECTION ( 'NONE',  ( 0.9609149988134843001, -0.1028163501681632064, 0.2570431154366505933 ) ) ;
#11663=CARTESIAN_POINT ( 'NONE',  ( 70.19189222814998175, -62.26243369865490251, -38.10776559704283528 ) ) ;
#11678=EDGE_LOOP ( 'NONE', ( #35436, #36749, #42195, #7786 ) ) ;
#11679=EDGE_CURVE ( 'NONE', #42441, #39438, #4294, .T. ) ;
#11685=ORIENTED_EDGE ( 'NONE', *, *, #3931, .F. ) ;
#11699=AXIS2_PLACEMENT_3D ( 'NONE', #27661, #34033, #13303 ) ;
#11704=VERTEX_POINT ( 'NONE', #25289 ) ;
#11706=EDGE_CURVE ( 'NONE', #33236, #27364, #33476, .T. ) ;
#11741=EDGE_CURVE ( 'NONE', #10810, #35134, #8182, .T. ) ;
#11744=AXIS2_PLACEMENT_3D ( 'NONE', #29721, #1453, #19011 ) ;
#11747=AXIS2_PLACEMENT_3D ( 'NONE', #34529, #24297, #31121 ) ;
#11764=DIRECTION ( 'NONE',  ( 0.9609149988134837450, -0.1028163501681639419, 0.2570431154366518145 ) ) ;
#11772=CARTESIAN_POINT ( 'NONE',  ( 73.07463722459043254, -61.07442264524582498, -36.73805742556071152 ) ) ;
#11791=EDGE_CURVE ( 'NONE', #35800, #29125, #21845, .T. ) ;
#11808=DIRECTION ( 'NONE',  ( 0.9609149988134837450, -0.1028163501681639419, 0.2570431154366518145 ) ) ;
#11823=ORIENTED_EDGE ( 'NONE', *, *, #11485, .T. ) ;
#11857=AXIS2_PLACEMENT_3D ( 'NONE', #28055, #20545, #3431 ) ;
#11858=CARTESIAN_POINT ( 'NONE',  ( 70.19189222814998175, -51.48119552555760947, -33.79530790927901052 ) ) ;
#11885=ORIENTED_EDGE ( 'NONE', *, *, #40181, .F. ) ;
#11895=ORIENTED_EDGE ( 'NONE', *, *, #23080, .F. ) ;
#11921=VERTEX_POINT ( 'NONE', #44203 ) ;
#11925=AXIS2_PLACEMENT_3D ( 'NONE', #42679, #42902, #10773 ) ;
#11974=CARTESIAN_POINT ( 'NONE',  ( 70.19189222814998175, -52.61716011954800365, -34.24968978710501943 ) ) ;
#12017=VECTOR ( 'NONE', #44005, 1000.000000000000227 ) ;
#12020=SHAPE_DEFINITION_REPRESENTATION ( #7751, #10805 ) ;
#12042=AXIS2_PLACEMENT_3D ( 'NONE', #7041, #7702, #17748 ) ;
#12053=ORIENTED_EDGE ( 'NONE', *, *, #28168, .T. ) ;
#12059=CARTESIAN_POINT ( 'NONE',  ( 70.19189222814998175, -57.25954915413987578, -36.10662921840084749 ) ) ;
#12068=ORIENTED_EDGE ( 'NONE', *, *, #11791, .T. ) ;
#12084=DIRECTION ( 'NONE',  ( 0.7871354856660198740, 0.4483307682966886643, 0.4235767337848242442 ) ) ;
#12088=VECTOR ( 'NONE', #43603, 1000.000000000000114 ) ;
#12089=DIRECTION ( 'NONE',  ( -0.000000000000000000, -0.9284778069183721172, -0.3713878862591650232 ) ) ;
#12108=AXIS2_PLACEMENT_3D ( 'NONE', #11198, #5912, #26454 ) ;
#12115=DIRECTION ( 'NONE',  ( -0.9609149988134837450, 0.1028163501681639419, -0.2570431154366518145 ) ) ;
#12140=AXIS2_PLACEMENT_3D ( 'NONE', #6146, #31210, #6381 ) ;
#12149=LINE ( 'NONE', #39511, #12088 ) ;
#12164=VERTEX_POINT ( 'NONE', #15929 ) ;
#12167=CARTESIAN_POINT ( 'NONE',  ( 71.02242295334774269, -54.12449018237889220, -37.95742420651561133 ) ) ;
#12172=VECTOR ( 'NONE', #19681, 1000.000000000000227 ) ;
#12184=VERTEX_POINT ( 'NONE', #9084 ) ;
#12185=AXIS2_PLACEMENT_3D ( 'NONE', #8161, #5403, #1309 ) ;
#12243=CARTESIAN_POINT ( 'NONE',  ( 70.19189222814998175, -53.54563792646638376, -34.62107767336419073 ) ) ;
#12252=EDGE_CURVE ( 'NONE', #10287, #13764, #30847, .T. ) ;
#12257=CYLINDRICAL_SURFACE ( 'NONE', #32259, 3.000000000000001776 ) ;
#12264=CIRCLE ( 'NONE', #24028, 2.445500000000004448 ) ;
#12303=EDGE_CURVE ( 'NONE', #21214, #39653, #19914, .T. ) ;
#12307=DIRECTION ( 'NONE',  ( -0.000000000000000000, -0.9284778069183718952, -0.3713878862591649677 ) ) ;
#12314=ORIENTED_EDGE ( 'NONE', *, *, #935, .T. ) ;
#12335=CARTESIAN_POINT ( 'NONE',  ( 71.02242295334774269, -50.41057895470540728, -36.47187266147894746 ) ) ;
#12346=LINE ( 'NONE', #36936, #32981 ) ;
#12358=ADVANCED_FACE ( 'NONE', ( #26978 ), #40898, .T. ) ;
#12362=EDGE_LOOP ( 'NONE', ( #4780, #40621, #13263, #39241, #7111, #12809 ) ) ;
#12363=CONICAL_SURFACE ( 'NONE', #18179, 2.999999999999999556, 0.9599310885968830309 ) ;
#12375=AXIS2_PLACEMENT_3D ( 'NONE', #42185, #21649, #10727 ) ;
#12376=DIRECTION ( 'NONE',  ( 0.9609149988134837450, -0.1028163501681639419, 0.2570431154366518145 ) ) ;
#12377=DIRECTION ( 'NONE',  ( -0.000000000000000000, -0.9284778069183718952, -0.3713878862591649677 ) ) ;
#12380=EDGE_CURVE ( 'NONE', #41822, #18421, #10246, .T. ) ;
#12386=ORIENTED_EDGE ( 'NONE', *, *, #40719, .T. ) ;
#12427=FACE_OUTER_BOUND ( 'NONE', #8808, .T. ) ;
#12429=AXIS2_PLACEMENT_3D ( 'NONE', #12690, #18841, #22042 ) ;
#12448=CARTESIAN_POINT ( 'NONE',  ( 72.54180985774836188, -52.30061520688905574, -33.39389990939168484 ) ) ;
#12456=AXIS2_PLACEMENT_3D ( 'NONE', #18335, #15984, #15140 ) ;
#12489=CARTESIAN_POINT ( 'NONE',  ( 73.07463722459043254, -56.43203361065396706, -34.88111799426488346 ) ) ;
#12494=CIRCLE ( 'NONE', #38701, 2.999999999999999556 ) ;
#12526=DIRECTION ( 'NONE',  ( -0.6937550123170076466, 0.2674776663120608799, -0.6686999932026935767 ) ) ;
#12554=EDGE_CURVE ( 'NONE', #33002, #42672, #23459, .T. ) ;
#12575=EDGE_LOOP ( 'NONE', ( #15745, #8416, #40910, #10951, #7777 ) ) ;
#12579=FACE_OUTER_BOUND ( 'NONE', #14901, .T. ) ;
#12584=VERTEX_POINT ( 'NONE', #11030 ) ;
#12598=ORIENTED_EDGE ( 'NONE', *, *, #8387, .F. ) ;
#12633=AXIS2_PLACEMENT_3D ( 'NONE', #8375, #25259, #32080 ) ;
#12650=ORIENTED_EDGE ( 'NONE', *, *, #11649, .T. ) ;
#12690=CARTESIAN_POINT ( 'NONE',  ( 70.19189222814998175, -55.76308905022629858, -35.50805039322867884 ) ) ;
#12706=ORIENTED_EDGE ( 'NONE', *, *, #19437, .F. ) ;
#12709=CARTESIAN_POINT ( 'NONE',  ( 71.02242295334774269, -99.02728775972636299, -55.91838671430374319 ) ) ;
#12741=ORIENTED_EDGE ( 'NONE', *, *, #25298, .F. ) ;
#12742=CARTESIAN_POINT ( 'NONE',  ( 70.19189222814998175, -51.12070001563444066, -33.65111096193285078 ) ) ;
#12749=( NAMED_UNIT ( * ) SI_UNIT ( $, .STERADIAN. ) SOLID_ANGLE_UNIT ( ) );
#12763=CIRCLE ( 'NONE', #20056, 2.999999999999999556 ) ;
#12766=DIRECTION ( 'NONE',  ( -0.000000000000000000, -0.9284778069183718952, -0.3713878862591649677 ) ) ;
#12768=CARTESIAN_POINT ( 'NONE',  ( 70.19189222814998175, -56.33107134722149567, -35.73524133214168330 ) ) ;
#12787=DIRECTION ( 'NONE',  ( -0.9609149988134837450, 0.1028163501681639419, -0.2570431154366518145 ) ) ;
#12796=EDGE_CURVE ( 'NONE', #25152, #26514, #11490, .T. ) ;
#12809=ORIENTED_EDGE ( 'NONE', *, *, #28101, .F. ) ;
#12810=AXIS2_PLACEMENT_3D ( 'NONE', #16528, #41154, #10361 ) ;
#12818=ADVANCED_FACE ( 'NONE', ( #21289 ), #39523, .T. ) ;
#12826=AXIS2_PLACEMENT_3D ( 'NONE', #5374, #1946, #19059 ) ;
#12831=CONICAL_SURFACE ( 'NONE', #38288, 2.445500000000004448, 0.9599310885968757034 ) ;
#12836=DIRECTION ( 'NONE',  ( 0.9609149988134843001, -0.1028163501681632064, 0.2570431154366505933 ) ) ;
#12837=CARTESIAN_POINT ( 'NONE',  ( 70.19189222814998175, -57.05206236706784040, -36.02363522683400276 ) ) ;
#12872=AXIS2_PLACEMENT_3D ( 'NONE', #35278, #194, #14110 ) ;
#12877=VERTEX_POINT ( 'NONE', #13011 ) ;
#12910=DIRECTION ( 'NONE',  ( -0.2768435750659241079, -0.3568721902840695792, 0.8921882507333129819 ) ) ;
#12929=ORIENTED_EDGE ( 'NONE', *, *, #38158, .T. ) ;
#12940=CARTESIAN_POINT ( 'NONE',  ( 72.54180985774836188, -54.15757082072580175, -34.13667568191001322 ) ) ;
#12947=DIRECTION ( 'NONE',  ( 1.387778780781445676E-17, -0.9284778069183720062, -0.3713878862591650232 ) ) ;
#12973=ORIENTED_EDGE ( 'NONE', *, *, #40399, .F. ) ;
#12993=FACE_OUTER_BOUND ( 'NONE', #20140, .T. ) ;
#12994=DIRECTION ( 'NONE',  ( -0.000000000000000000, -0.9284778069183721172, -0.3713878862591650232 ) ) ;
#13011=CARTESIAN_POINT ( 'NONE',  ( 71.02242295334774269, -59.69535702388913023, -40.18575152407060358 ) ) ;
#13023=CARTESIAN_POINT ( 'NONE',  ( 72.54180985774836188, -59.72843766223603268, -36.36500299946500547 ) ) ;
#13048=EDGE_CURVE ( 'NONE', #30068, #14242, #24846, .T. ) ;
#13061=EDGE_CURVE ( 'NONE', #19163, #4387, #17559, .T. ) ;
#13068=ORIENTED_EDGE ( 'NONE', *, *, #21309, .T. ) ;
#13089=AXIS2_PLACEMENT_3D ( 'NONE', #33331, #2105, #4633 ) ;
#13092=EDGE_LOOP ( 'NONE', ( #23292, #14800, #16661, #26716, #5398, #33309 ) ) ;
#13098=CARTESIAN_POINT ( 'NONE',  ( 69.48815586033239811, -68.74046964786722924, -38.06815038123374251 ) ) ;
#13108=DIRECTION ( 'NONE',  ( 0.9609149988134837450, -0.1028163501681639419, 0.2570431154366518145 ) ) ;
#13113=CARTESIAN_POINT ( 'NONE',  ( 70.19189222814998175, -60.97346038181336070, -37.59218076343751136 ) ) ;
#13119=CARTESIAN_POINT ( 'NONE',  ( 73.07463722459043254, -54.78256478388924933, -34.22133621331339981 ) ) ;
#13122=EDGE_LOOP ( 'NONE', ( #28798, #33500, #9437, #1937, #18351 ) ) ;
#13132=CYLINDRICAL_SURFACE ( 'NONE', #9170, 3.000000000000001776 ) ;
#13162=DIRECTION ( 'NONE',  ( 0.9609149988134843001, -0.1028163501681632064, 0.2570431154366505933 ) ) ;
#13172=VECTOR ( 'NONE', #27101, 1000.000000000000227 ) ;
#13192=ORIENTED_EDGE ( 'NONE', *, *, #38276, .T. ) ;
#13226=FACE_OUTER_BOUND ( 'NONE', #39481, .T. ) ;
#13239=CIRCLE ( 'NONE', #38692, 2.999999999999999556 ) ;
#13245=CARTESIAN_POINT ( 'NONE',  ( 69.36136150295220659, -54.40876771024655056, -31.86151892959740550 ) ) ;
#13250=DIRECTION ( 'NONE',  ( 0.7871354856660167654, -0.6167752151498625546, -0.002461946824136807422 ) ) ;
#13251=VERTEX_POINT ( 'NONE', #10707 ) ;
#13263=ORIENTED_EDGE ( 'NONE', *, *, #28400, .T. ) ;
#13294=VERTEX_POINT ( 'NONE', #25059 ) ;
#13303=DIRECTION ( 'NONE',  ( -0.2768435750659241079, -0.3568721902840695792, 0.8921882507333129819 ) ) ;
#13318=EDGE_CURVE ( 'NONE', #11704, #17071, #876, .T. ) ;
#13320=CIRCLE ( 'NONE', #38765, 2.999999999999999556 ) ;
#13352=ORIENTED_EDGE ( 'NONE', *, *, #44006, .T. ) ;
#13362=DIRECTION ( 'NONE',  ( 0.2407039305251456596, -0.3604685577742790525, 0.9011792478113757054 ) ) ;
#13382=VERTEX_POINT ( 'NONE', #32774 ) ;
#13393=DIRECTION ( 'NONE',  ( 0.9609149988134843001, -0.1028163501681632064, 0.2570431154366505933 ) ) ;
#13402=FACE_OUTER_BOUND ( 'NONE', #23914, .T. ) ;
#13413=CIRCLE ( 'NONE', #19223, 2.999999999999999556 ) ;
#13450=DIRECTION ( 'NONE',  ( -0.000000000000000000, -0.9284778069183721172, -0.3713878862591650232 ) ) ;
#13453=LINE ( 'NONE', #25500, #37619 ) ;
#13462=ORIENTED_EDGE ( 'NONE', *, *, #33087, .F. ) ;
#13467=DIRECTION ( 'NONE',  ( -0.000000000000000000, -0.9284778069183721172, -0.3713878862591650232 ) ) ;
#13484=FACE_OUTER_BOUND ( 'NONE', #22578, .T. ) ;
#13491=ORIENTED_EDGE ( 'NONE', *, *, #12303, .T. ) ;
#13498=ORIENTED_EDGE ( 'NONE', *, *, #26991, .T. ) ;
#13527=CARTESIAN_POINT ( 'NONE',  ( 70.19189222814998175, -62.62292920857806422, -38.25196254438899501 ) ) ;
#13577=CARTESIAN_POINT ( 'NONE',  ( 70.19189222814998175, -100.0979043305785581, -53.24182196210380624 ) ) ;
#13579=AXIS2_PLACEMENT_3D ( 'NONE', #10866, #28642, #20907 ) ;
#13588=CARTESIAN_POINT ( 'NONE',  ( 69.36136150295220659, -62.97255475958395010, -35.28700389749673860 ) ) ;
#13620=DIRECTION ( 'NONE',  ( -0.000000000000000000, -0.9284778069183721172, -0.3713878862591650232 ) ) ;
#13636=TOROIDAL_SURFACE ( 'NONE', #15092, 3.250000000000000000, 0.2500000000000000000 ) ;
#13668=CARTESIAN_POINT ( 'NONE',  ( 70.19189222814998175, -100.0979043305785581, -53.24182196210380624 ) ) ;
#13682=ORIENTED_EDGE ( 'NONE', *, *, #43991, .T. ) ;
#13697=LINE ( 'NONE', #3423, #17022 ) ;
#13707=ADVANCED_FACE ( 'NONE', ( #22201 ), #21911, .T. ) ;
#13723=APPLICATION_CONTEXT ( 'automotive_design' ) ;
#13754=ORIENTED_EDGE ( 'NONE', *, *, #8059, .F. ) ;
#13764=VERTEX_POINT ( 'NONE', #28827 ) ;
#13789=DIRECTION ( 'NONE',  ( 0.7871354856660167654, -0.6167752151498625546, -0.002461946824136807422 ) ) ;
#13807=CARTESIAN_POINT ( 'NONE',  ( 67.37136766119182596, -67.53150897494617766, -41.09057840265009531 ) ) ;
#13866=CIRCLE ( 'NONE', #26986, 2.445500000000004448 ) ;
#13874=ORIENTED_EDGE ( 'NONE', *, *, #13061, .F. ) ;
#13917=AXIS2_PLACEMENT_3D ( 'NONE', #7491, #21408, #21856 ) ;
#13919=DIRECTION ( 'NONE',  ( 0.000000000000000000, 0.9284778069183720062, 0.3713878862591650232 ) ) ;
#13937=ORIENTED_EDGE ( 'NONE', *, *, #1919, .T. ) ;
#13944=DIRECTION ( 'NONE',  ( 0.7871354856660198740, 0.4483307682966886643, 0.4235767337848242442 ) ) ;
#13959=CARTESIAN_POINT ( 'NONE',  ( 70.19189222814998175, -60.40547808481815650, -37.36498982452450690 ) ) ;
#13972=DIRECTION ( 'NONE',  ( 0.9609149988134837450, -0.1028163501681639419, 0.2570431154366518145 ) ) ;
#14005=DIRECTION ( 'NONE',  ( -0.000000000000000000, -0.9284778069183718952, -0.3713878862591649677 ) ) ;
#14023=CARTESIAN_POINT ( 'NONE',  ( 70.19189222814998175, -65.04786711941001442, -39.22192925582032785 ) ) ;
#14046=CARTESIAN_POINT ( 'NONE',  ( 70.19189222814998175, -100.0979043305785581, -53.24182196210380624 ) ) ;
#14067=CIRCLE ( 'NONE', #16256, 5.000000000000002665 ) ;
#14081=LINE ( 'NONE', #24131, #21356 ) ;
#14093=ORIENTED_EDGE ( 'NONE', *, *, #31868, .F. ) ;
#14105=LINE ( 'NONE', #35044, #25131 ) ;
#14110=DIRECTION ( 'NONE',  ( 0.9609149988134837450, -0.1028163501681639419, 0.2570431154366518145 ) ) ;
#14116=ORIENTED_EDGE ( 'NONE', *, *, #35623, .F. ) ;
#14123=ORIENTED_EDGE ( 'NONE', *, *, #11679, .T. ) ;
#14126=DIRECTION ( 'NONE',  ( 1.387778780781445676E-17, -0.9284778069183720062, -0.3713878862591650232 ) ) ;
#14161=DIRECTION ( 'NONE',  ( -0.000000000000000000, -0.9284778069183720062, -0.3713878862591650232 ) ) ;
#14169=ORIENTED_EDGE ( 'NONE', *, *, #2761, .F. ) ;
#14180=LINE ( 'NONE', #17607, #37978 ) ;
#14184=DIRECTION ( 'NONE',  ( -0.9609149988134837450, 0.1028163501681639419, -0.2570431154366518145 ) ) ;
#14189=AXIS2_PLACEMENT_3D ( 'NONE', #20465, #13620, #34346 ) ;
#14203=VECTOR ( 'NONE', #23146, 1000.000000000000227 ) ;
#14211=ORIENTED_EDGE ( 'NONE', *, *, #23080, .T. ) ;
#14219=AXIS2_PLACEMENT_3D ( 'NONE', #7985, #38760, #35788 ) ;
#14226=ORIENTED_EDGE ( 'NONE', *, *, #4145, .T. ) ;
#14232=VERTEX_POINT ( 'NONE', #36796 ) ;
#14242=VERTEX_POINT ( 'NONE', #29298 ) ;
#14255=CONICAL_SURFACE ( 'NONE', #43352, 2.445500000000004448, 0.9599310885968757034 ) ;
#14269=DIRECTION ( 'NONE',  ( -0.2768435750659241079, -0.3568721902840695792, 0.8921882507333129819 ) ) ;
#14273=DIRECTION ( 'NONE',  ( -0.000000000000000000, -0.9284778069183721172, -0.3713878862591650232 ) ) ;
#14274=CARTESIAN_POINT ( 'NONE',  ( 70.19189222814998175, -53.54563792646638376, -34.62107767336419073 ) ) ;
#14284=ORIENTED_EDGE ( 'NONE', *, *, #18912, .F. ) ;
#14306=CARTESIAN_POINT ( 'NONE',  ( 71.02242295334774269, -58.97436600404279972, -39.89735762937828412 ) ) ;
#14309=EDGE_CURVE ( 'NONE', #29611, #13251, #3005, .T. ) ;
#14311=CIRCLE ( 'NONE', #1187, 2.445500000000004448 ) ;
#14324=ORIENTED_EDGE ( 'NONE', *, *, #27018, .F. ) ;
#14344=DIRECTION ( 'NONE',  ( -0.000000000000000000, -0.9284778069183718952, -0.3713878862591649677 ) ) ;
#14345=DIRECTION ( 'NONE',  ( 0.9609149988134837450, -0.1028163501681639419, 0.2570431154366518145 ) ) ;
#14346=DIRECTION ( 'NONE',  ( -0.2768435750659253847, -0.3568721902840677473, 0.8921882507333133150 ) ) ;
#14368=ORIENTED_EDGE ( 'NONE', *, *, #40911, .F. ) ;
#14391=LINE ( 'NONE', #38540, #21097 ) ;
#14413=ORIENTED_EDGE ( 'NONE', *, *, #17762, .T. ) ;
#14423=EDGE_CURVE ( 'NONE', #37456, #26292, #18303, .T. ) ;
#14429=ADVANCED_FACE ( 'NONE', ( #87 ), #41608, .T. ) ;
#14436=CIRCLE ( 'NONE', #21005, 2.541999999999999371 ) ;
#14441=LINE ( 'NONE', #10802, #33936 ) ;
#14508=VERTEX_POINT ( 'NONE', #30429 ) ;
#14510=EDGE_CURVE ( 'NONE', #16083, #3126, #21946, .T. ) ;
#14515=DIRECTION ( 'NONE',  ( 0.9609149988134843001, -0.1028163501681632064, 0.2570431154366505933 ) ) ;
#14542=EDGE_CURVE ( 'NONE', #16121, #25152, #1561, .T. ) ;
#14550=CARTESIAN_POINT ( 'NONE',  ( 71.02242295334774269, -58.04588819712443382, -39.52596974311911993 ) ) ;
#14575=DIRECTION ( 'NONE',  ( -0.000000000000000000, -0.9284778069183721172, -0.3713878862591650232 ) ) ;
#14582=CARTESIAN_POINT ( 'NONE',  ( 73.01241679510815175, -68.13509210538408922, -39.58160742654554554 ) ) ;
#14609=CARTESIAN_POINT ( 'NONE',  ( 70.19189222814998175, -57.05206236706784040, -36.02363522683400276 ) ) ;
#14624=VECTOR ( 'NONE', #14344, 1000.000000000000227 ) ;
#14715=DIRECTION ( 'NONE',  ( -0.000000000000000000, -0.9284778069183721172, -0.3713878862591650232 ) ) ;
#14723=DIRECTION ( 'NONE',  ( -0.000000000000000000, -0.9284778069183721172, -0.3713878862591650232 ) ) ;
#14756=VERTEX_POINT ( 'NONE', #32631 ) ;
#14770=EDGE_LOOP ( 'NONE', ( #23221, #31978, #21629, #7018, #29437 ) ) ;
#14774=DIRECTION ( 'NONE',  ( -0.000000000000000000, -0.9284778069183718952, -0.3713878862591649677 ) ) ;
#14781=DIRECTION ( 'NONE',  ( -0.9609149988134837450, 0.1028163501681645109, -0.2570431154366520921 ) ) ;
#14784=AXIS2_PLACEMENT_3D ( 'NONE', #27817, #20754, #17335 ) ;
#14792=ORIENTED_EDGE ( 'NONE', *, *, #8059, .T. ) ;
#14795=CARTESIAN_POINT ( 'NONE',  ( 69.36136150295220659, -101.1685209014307674, -50.56525720990386219 ) ) ;
#14797=DIRECTION ( 'NONE',  ( -0.000000000000000000, -0.9284778069183721172, -0.3713878862591650232 ) ) ;
#14800=ORIENTED_EDGE ( 'NONE', *, *, #22250, .T. ) ;
#14805=EDGE_CURVE ( 'NONE', #14242, #35800, #13239, .T. ) ;
#14820=ORIENTED_EDGE ( 'NONE', *, *, #26999, .F. ) ;
#14828=DIRECTION ( 'NONE',  ( -0.000000000000000000, -0.9284778069183721172, -0.3713878862591650232 ) ) ;
#14855=DIRECTION ( 'NONE',  ( -0.000000000000000000, -0.9284778069183720062, -0.3713878862591650232 ) ) ;
#14871=CARTESIAN_POINT ( 'NONE',  ( 70.19189222814998175, -54.47411573338475677, -34.99246555962335492 ) ) ;
#14877=EDGE_CURVE ( 'NONE', #19823, #44794, #28333, .T. ) ;
#14883=CONICAL_SURFACE ( 'NONE', #19994, 2.445500000000004448, 0.9599310885968757034 ) ;
#14901=EDGE_LOOP ( 'NONE', ( #19416, #663, #20033, #1853, #37146, #993 ) ) ;
#14904=DIRECTION ( 'NONE',  ( -0.000000000000000000, -0.9284778069183718952, -0.3713878862591649677 ) ) ;
#14953=CARTESIAN_POINT ( 'NONE',  ( 71.57611010347959279, -68.55582966742440476, -45.79978146116413029 ) ) ;
#14981=CONICAL_SURFACE ( 'NONE', #20102, 2.445500000000004448, 0.9599310885968757034 ) ;
#14994=EDGE_CURVE ( 'NONE', #16741, #36562, #37257, .T. ) ;
#14997=DIRECTION ( 'NONE',  ( -0.2768435750659243300, -0.3568721902840689131, 0.8921882507333129819 ) ) ;
#14999=CARTESIAN_POINT ( 'NONE',  ( 70.19189222814998175, -58.18802696105826300, -36.47801710466001879 ) ) ;
#15016=ADVANCED_FACE ( 'NONE', ( #16911 ), #31686, .T. ) ;
#15032=AXIS2_PLACEMENT_3D ( 'NONE', #27304, #23202, #3123 ) ;
#15040=LINE ( 'NONE', #28950, #23780 ) ;
#15070=VERTEX_POINT ( 'NONE', #24195 ) ;
#15080=FACE_OUTER_BOUND ( 'NONE', #7981, .T. ) ;
#15092=AXIS2_PLACEMENT_3D ( 'NONE', #16808, #20449, #9963 ) ;
#15117=DIRECTION ( 'NONE',  ( -0.000000000000000000, -0.9284778069183721172, -0.3713878862591650232 ) ) ;
#15128=DIRECTION ( 'NONE',  ( 0.9609149988134837450, -0.1028163501681639419, 0.2570431154366518145 ) ) ;
#15140=DIRECTION ( 'NONE',  ( 0.9609149988134843001, -0.1028163501681632064, 0.2570431154366505933 ) ) ;
#15202=DIRECTION ( 'NONE',  ( -0.000000000000000000, -0.9284778069183721172, -0.3713878862591650232 ) ) ;
#15244=VERTEX_POINT ( 'NONE', #10953 ) ;
#15258=FACE_OUTER_BOUND ( 'NONE', #38026, .T. ) ;
#15276=DIRECTION ( 'NONE',  ( -0.9609149988134837450, 0.1028163501681639419, -0.2570431154366518145 ) ) ;
#15297=ORIENTED_EDGE ( 'NONE', *, *, #17407, .T. ) ;
#15300=CARTESIAN_POINT ( 'NONE',  ( 70.19189222814998175, -67.83330054016514055, -40.33609291459782753 ) ) ;
#15313=DIRECTION ( 'NONE',  ( 0.9609149988134837450, -0.1028163501681639419, 0.2570431154366518145 ) ) ;
#15317=ORIENTED_EDGE ( 'NONE', *, *, #24542, .F. ) ;
#15329=ORIENTED_EDGE ( 'NONE', *, *, #15945, .T. ) ;
#15338=CARTESIAN_POINT ( 'NONE',  ( 71.02242295334774269, -99.02728775972636299, -55.91838671430374319 ) ) ;
#15356=ORIENTED_EDGE ( 'NONE', *, *, #8613, .F. ) ;
#15398=DIRECTION ( 'NONE',  ( -0.000000000000000000, -0.9284778069183720062, -0.3713878862591650232 ) ) ;
#15455=DIRECTION ( 'NONE',  ( -0.000000000000000000, -0.9284778069183721172, -0.3713878862591650232 ) ) ;
#15465=EDGE_LOOP ( 'NONE', ( #26416, #10703, #730, #22192, #31656 ) ) ;
#15474=ORIENTED_EDGE ( 'NONE', *, *, #43991, .F. ) ;
#15484=DIRECTION ( 'NONE',  ( 0.9609149988134843001, -0.1028163501681632064, 0.2570431154366505933 ) ) ;
#15496=DIRECTION ( 'NONE',  ( 0.9609149988134837450, -0.1028163501681639419, 0.2570431154366518145 ) ) ;
#15506=AXIS2_PLACEMENT_3D ( 'NONE', #14046, #24097, #20227 ) ;
#15524=DIRECTION ( 'NONE',  ( 0.9609149988134837450, -0.1028163501681639419, 0.2570431154366518145 ) ) ;
#15546=ORIENTED_EDGE ( 'NONE', *, *, #31868, .T. ) ;
#15553=ORIENTED_EDGE ( 'NONE', *, *, #29229, .T. ) ;
#15568=DIRECTION ( 'NONE',  ( -0.000000000000000000, -0.9284778069183720062, -0.3713878862591650232 ) ) ;
#15574=CIRCLE ( 'NONE', #33026, 2.445500000000004448 ) ;
#15587=LINE ( 'NONE', #29489, #7549 ) ;
#15616=DIRECTION ( 'NONE',  ( 0.9609149988134837450, -0.1028163501681639419, 0.2570431154366518145 ) ) ;
#15622=EDGE_LOOP ( 'NONE', ( #29875, #41776, #35573, #35091, #3599, #18469 ) ) ;
#15683=AXIS2_PLACEMENT_3D ( 'NONE', #22292, #18649, #8611 ) ;
#15725=AXIS2_PLACEMENT_3D ( 'NONE', #4219, #11528, #800 ) ;
#15745=ORIENTED_EDGE ( 'NONE', *, *, #6423, .F. ) ;
#15751=EDGE_CURVE ( 'NONE', #28070, #32861, #33101, .T. ) ;
#15783=EDGE_LOOP ( 'NONE', ( #24740, #2210, #5748, #26623, #32557 ) ) ;
#15805=ORIENTED_EDGE ( 'NONE', *, *, #5330, .T. ) ;
#15840=EDGE_CURVE ( 'NONE', #15917, #38098, #43863, .T. ) ;
#15847=CARTESIAN_POINT ( 'NONE',  ( 70.19189222814998175, -53.33815113939435548, -34.53808368179734600 ) ) ;
#15851=CARTESIAN_POINT ( 'NONE',  ( 69.48536631248848039, -69.56066907060868232, -44.09544185076553191 ) ) ;
#15882=DIRECTION ( 'NONE',  ( -0.000000000000000000, -0.9284778069183718952, -0.3713878862591649677 ) ) ;
#15884=UNCERTAINTY_MEASURE_WITH_UNIT (LENGTH_MEASURE( 1.000000000000000082E-05 ), #23883, 'distance_accuracy_value', 'NONE');
#15885=CARTESIAN_POINT ( 'NONE',  ( 70.19189222814998175, -57.62004466406304459, -36.25082616574700722 ) ) ;
#15886=EDGE_CURVE ( 'NONE', #3470, #31689, #9656, .T. ) ;
#15897=CARTESIAN_POINT ( 'NONE',  ( 70.19189222814998175, -100.0979043305785581, -53.24182196210380624 ) ) ;
#15898=ORIENTED_EDGE ( 'NONE', *, *, #21087, .F. ) ;
#15917=VERTEX_POINT ( 'NONE', #44755 ) ;
#15929=CARTESIAN_POINT ( 'NONE',  ( 67.30914723170953096, -58.60056893040009385, -37.53754034566229336 ) ) ;
#15945=EDGE_CURVE ( 'NONE', #29611, #40557, #34242, .T. ) ;
#15984=DIRECTION ( 'NONE',  ( -0.000000000000000000, -0.9284778069183720062, -0.3713878862591650232 ) ) ;
#16033=PLANE ( 'NONE',  #42921 ) ;
#16048=DIRECTION ( 'NONE',  ( 0.7871354856660167654, -0.6167752151498625546, -0.002461946824136807422 ) ) ;
#16052=ORIENTED_EDGE ( 'NONE', *, *, #29888, .T. ) ;
#16083=VERTEX_POINT ( 'NONE', #35345 ) ;
#16085=DIRECTION ( 'NONE',  ( 0.7871354856660167654, -0.6167752151498625546, -0.002461946824136807422 ) ) ;
#16094=DIRECTION ( 'NONE',  ( 0.2768435750659360983, 0.3568721902840809590, -0.8921882507333046552 ) ) ;
#16098=CARTESIAN_POINT ( 'NONE',  ( 70.89841814381148311, -71.67679885123182260, -38.80507129598510119 ) ) ;
#16121=VERTEX_POINT ( 'NONE', #8456 ) ;
#16156=CARTESIAN_POINT ( 'NONE',  ( 70.89841814381148311, -68.89136543047671069, -37.69090763720760151 ) ) ;
#16174=VECTOR ( 'NONE', #28704, 1000.000000000000227 ) ;
#16186=LINE ( 'NONE', #40352, #12017 ) ;
#16191=FACE_OUTER_BOUND ( 'NONE', #3799, .T. ) ;
#16251=FACE_OUTER_BOUND ( 'NONE', #32364, .T. ) ;
#16256=AXIS2_PLACEMENT_3D ( 'NONE', #41256, #16624, #40794 ) ;
#16259=AXIS2_PLACEMENT_3D ( 'NONE', #23839, #40938, #482 ) ;
#16263=ORIENTED_EDGE ( 'NONE', *, *, #1047, .T. ) ;
#16265=DIRECTION ( 'NONE',  ( 0.9609149988134837450, -0.1028163501681639419, 0.2570431154366518145 ) ) ;
#16306=ORIENTED_EDGE ( 'NONE', *, *, #16975, .T. ) ;
#16309=DIRECTION ( 'NONE',  ( -0.000000000000000000, -0.9284778069183721172, -0.3713878862591650232 ) ) ;
#16324=DIRECTION ( 'NONE',  ( -0.2768435750659241079, -0.3568721902840695792, 0.8921882507333129819 ) ) ;
#16325=LINE ( 'NONE', #34527, #34703 ) ;
#16347=ORIENTED_EDGE ( 'NONE', *, *, #7871, .T. ) ;
#16363=EDGE_LOOP ( 'NONE', ( #36882, #3034, #34835, #32341, #43710 ) ) ;
#16384=CARTESIAN_POINT ( 'NONE',  ( 67.30914723170953096, -57.67209112348172084, -37.16615245940312207 ) ) ;
#16385=AXIS2_PLACEMENT_3D ( 'NONE', #43724, #15455, #36856 ) ;
#16393=CARTESIAN_POINT ( 'NONE',  ( 67.84197459855160162, -60.15404070048191443, -37.99358876332483703 ) ) ;
#16400=CARTESIAN_POINT ( 'NONE',  ( 71.02242295334774269, -99.02728775972636299, -55.91838671430374319 ) ) ;
#16415=ADVANCED_FACE ( 'NONE', ( #25458 ), #19833, .T. ) ;
#16419=CARTESIAN_POINT ( 'NONE',  ( 71.57611010347959279, -63.26350616798967508, -43.68287050948689654 ) ) ;
#16444=ORIENTED_EDGE ( 'NONE', *, *, #38125, .T. ) ;
#16468=CARTESIAN_POINT ( 'NONE',  ( 72.54180985774836188, -56.01452643456254776, -34.87945145442834871 ) ) ;
#16491=VERTEX_POINT ( 'NONE', #11772 ) ;
#16500=CARTESIAN_POINT ( 'NONE',  ( 69.36136150295220659, -101.1685209014307674, -50.56525720990386219 ) ) ;
#16512=ORIENTED_EDGE ( 'NONE', *, *, #23236, .T. ) ;
#16513=CONICAL_SURFACE ( 'NONE', #25218, 2.999999999999999556, 0.9599310885968830309 ) ;
#16528=CARTESIAN_POINT ( 'NONE',  ( 70.19189222814998175, -55.76308905022629858, -35.50805039322867884 ) ) ;
#16536=ORIENTED_EDGE ( 'NONE', *, *, #21018, .F. ) ;
#16556=DIRECTION ( 'NONE',  ( -0.7871354856660202071, 0.6167752151498580027, 0.002461946824133919541 ) ) ;
#16563=CARTESIAN_POINT ( 'NONE',  ( 69.36136150295220659, -55.54473230423695185, -32.31590080742341797 ) ) ;
#16571=AXIS2_PLACEMENT_3D ( 'NONE', #7354, #10350, #31524 ) ;
#16573=ORIENTED_EDGE ( 'NONE', *, *, #42493, .F. ) ;
#16585=ADVANCED_FACE ( 'NONE', ( #22475 ), #34430, .T. ) ;
#16598=EDGE_LOOP ( 'NONE', ( #6398, #13352, #13874, #11435, #30586 ) ) ;
#16618=DIRECTION ( 'NONE',  ( -0.2768435750659266059, -0.3568721902840680249, 0.8921882507333128709 ) ) ;
#16624=DIRECTION ( 'NONE',  ( -0.000000000000000000, -0.9284778069183721172, -0.3713878862591650232 ) ) ;
#16661=ORIENTED_EDGE ( 'NONE', *, *, #8588, .T. ) ;
#16680=ORIENTED_EDGE ( 'NONE', *, *, #4956, .T. ) ;
#16686=ORIENTED_EDGE ( 'NONE', *, *, #14309, .T. ) ;
#16689=ADVANCED_BREP_SHAPE_REPRESENTATION ( '', ( #6206, #12375 ), #32596 ) ;
#16696=CONICAL_SURFACE ( 'NONE', #21066, 2.445500000000004448, 0.9599310885968757034 ) ;
#16713=ADVANCED_FACE ( 'NONE', ( #9475 ), #16782, .T. ) ;
#16722=DIRECTION ( 'NONE',  ( 0.9609149988134837450, -0.1028163501681639419, 0.2570431154366518145 ) ) ;
#16741=VERTEX_POINT ( 'NONE', #23851 ) ;
#16755=DIRECTION ( 'NONE',  ( 0.9609149988134837450, -0.1028163501681639419, 0.2570431154366518145 ) ) ;
#16758=VECTOR ( 'NONE', #39183, 1000.000000000000227 ) ;
#16759=DIRECTION ( 'NONE',  ( -0.000000000000000000, -0.9284778069183721172, -0.3713878862591650232 ) ) ;
#16774=AXIS2_PLACEMENT_3D ( 'NONE', #43493, #14774, #39161 ) ;
#16782=CYLINDRICAL_SURFACE ( 'NONE', #38796, 3.000000000000001776 ) ;
#16805=CIRCLE ( 'NONE', #27734, 2.999999999999999556 ) ;
#16808=CARTESIAN_POINT ( 'NONE',  ( 70.19189222814998175, -64.81574766768041229, -39.12908228425553858 ) ) ;
#16811=TOROIDAL_SURFACE ( 'NONE', #44462, 3.250000000000000000, 0.2500000000000000000 ) ;
#16853=ADVANCED_FACE ( 'NONE', ( #17440 ), #3080, .T. ) ;
#16868=AXIS2_PLACEMENT_3D ( 'NONE', #18505, #36263, #15524 ) ;
#16888=DIRECTION ( 'NONE',  ( -0.000000000000000000, -0.9284778069183721172, -0.3713878862591650232 ) ) ;
#16902=CIRCLE ( 'NONE', #18314, 2.999999999999999556 ) ;
#16911=FACE_OUTER_BOUND ( 'NONE', #43941, .T. ) ;
#16924=DIRECTION ( 'NONE',  ( 0.9609149988134837450, -0.1028163501681639419, 0.2570431154366518145 ) ) ;
#16969=VECTOR ( 'NONE', #37596, 1000.000000000000227 ) ;
#16975=EDGE_CURVE ( 'NONE', #22908, #21045, #25406, .T. ) ;
#16983=CONICAL_SURFACE ( 'NONE', #42457, 2.445500000000001339, 0.7853981633974680410 ) ;
#16984=DIRECTION ( 'NONE',  ( -0.000000000000000000, -0.9284778069183720062, -0.3713878862591650232 ) ) ;
#16985=CARTESIAN_POINT ( 'NONE',  ( 67.84197459855160162, -54.58317385897167640, -35.76526144576984478 ) ) ;
#16987=DIRECTION ( 'NONE',  ( -0.000000000000000000, -0.9284778069183718952, -0.3713878862591649677 ) ) ;
#16991=CARTESIAN_POINT ( 'NONE',  ( 70.19189222814998175, -60.76597359474132531, -37.50918677187066663 ) ) ;
#16992=EDGE_CURVE ( 'NONE', #9431, #20329, #9682, .T. ) ;
#16994=ORIENTED_EDGE ( 'NONE', *, *, #17855, .F. ) ;
#16995=LINE ( 'NONE', #44353, #3288 ) ;
#17017=CARTESIAN_POINT ( 'NONE',  ( 67.30914723170953096, -57.87957791055376333, -37.24914645096997390 ) ) ;
#17022=VECTOR ( 'NONE', #17340, 1000.000000000000227 ) ;
#17028=ORIENTED_EDGE ( 'NONE', *, *, #44578, .T. ) ;
#17036=LINE ( 'NONE', #30704, #31520 ) ;
#17071=VERTEX_POINT ( 'NONE', #107 ) ;
#17081=AXIS2_PLACEMENT_3D ( 'NONE', #4955, #28919, #7705 ) ;
#17085=ORIENTED_EDGE ( 'NONE', *, *, #37354, .T. ) ;
#17100=FACE_BOUND ( 'NONE', #17187, .T. ) ;
#17108=EDGE_LOOP ( 'NONE', ( #36270, #16686, #14226, #23401, #21021, #20451 ) ) ;
#17116=CARTESIAN_POINT ( 'NONE',  ( 67.84197459855160162, -54.58317385897167640, -35.76526144576984478 ) ) ;
#17130=DIRECTION ( 'NONE',  ( -0.9609149988134837450, 0.1028163501681639419, -0.2570431154366518145 ) ) ;
#17187=EDGE_LOOP ( 'NONE', ( #29798, #6651 ) ) ;
#17229=DIRECTION ( 'NONE',  ( 0.9609149988134837450, -0.1028163501681639419, 0.2570431154366518145 ) ) ;
#17254=DIRECTION ( 'NONE',  ( 0.7871354856660167654, -0.6167752151498625546, -0.002461946824136807422 ) ) ;
#17256=VECTOR ( 'NONE', #26809, 1000.000000000000227 ) ;
#17257=FACE_OUTER_BOUND ( 'NONE', #28819, .T. ) ;
#17313=VECTOR ( 'NONE', #1264, 999.9999999999998863 ) ;
#17330=FACE_OUTER_BOUND ( 'NONE', #22085, .T. ) ;
#17332=ORIENTED_EDGE ( 'NONE', *, *, #33350, .F. ) ;
#17335=DIRECTION ( 'NONE',  ( -0.2768435750659239414, -0.3568721902840664151, 0.8921882507333142032 ) ) ;
#17337=EDGE_CURVE ( 'NONE', #37423, #8341, #41730, .T. ) ;
#17340=DIRECTION ( 'NONE',  ( -0.000000000000000000, -0.9284778069183718952, -0.3713878862591649677 ) ) ;
#17345=AXIS2_PLACEMENT_3D ( 'NONE', #18604, #32495, #11764 ) ;
#17355=ADVANCED_FACE ( 'NONE', ( #435 ), #34633, .T. ) ;
#17363=EDGE_LOOP ( 'NONE', ( #17877, #6872, #18060, #28132 ) ) ;
#17388=CARTESIAN_POINT ( 'NONE',  ( 70.19189222814998175, -50.76020450571126474, -33.50691401458669105 ) ) ;
#17407=EDGE_CURVE ( 'NONE', #25810, #4027, #21326, .T. ) ;
#17408=CARTESIAN_POINT ( 'NONE',  ( 73.01241679510815175, -70.92052552613920113, -40.69577108532303811 ) ) ;
#17417=ORIENTED_EDGE ( 'NONE', *, *, #1622, .T. ) ;
#17432=ORIENTED_EDGE ( 'NONE', *, *, #6097, .F. ) ;
#17434=AXIS2_PLACEMENT_3D ( 'NONE', #24502, #18102, #38386 ) ;
#17440=FACE_OUTER_BOUND ( 'NONE', #17108, .T. ) ;
#17442=DIRECTION ( 'NONE',  ( -0.000000000000000000, -0.9284778069183721172, -0.3713878862591650232 ) ) ;
#17464=DIRECTION ( 'NONE',  ( -0.000000000000000000, -0.9284778069183721172, -0.3713878862591650232 ) ) ;
#17479=EDGE_LOOP ( 'NONE', ( #38889, #31959, #24492, #36431, #32736 ) ) ;
#17493=CARTESIAN_POINT ( 'NONE',  ( 70.19189222814998175, -61.90193818873174791, -37.96356864969668266 ) ) ;
#17500=CARTESIAN_POINT ( 'NONE',  ( 70.19189222814998175, -50.70706315265230302, -33.48565765860439569 ) ) ;
#17502=AXIS2_PLACEMENT_3D ( 'NONE', #19371, #12994, #8886 ) ;
#17508=EDGE_CURVE ( 'NONE', #43489, #17518, #27886, .T. ) ;
#17518=VERTEX_POINT ( 'NONE', #26977 ) ;
#17521=AXIS2_PLACEMENT_3D ( 'NONE', #10334, #27210, #24237 ) ;
#17524=FACE_OUTER_BOUND ( 'NONE', #13122, .T. ) ;
#17532=AXIS2_PLACEMENT_3D ( 'NONE', #25774, #1584, #5456 ) ;
#17533=EDGE_CURVE ( 'NONE', #3126, #219, #27915, .T. ) ;
#17555=ORIENTED_EDGE ( 'NONE', *, *, #25940, .F. ) ;
#17559=CIRCLE ( 'NONE', #13917, 2.999999999999999556 ) ;
#17579=ORIENTED_EDGE ( 'NONE', *, *, #12303, .F. ) ;
#17587=DIRECTION ( 'NONE',  ( 0.000000000000000000, 0.9284778069183718952, 0.3713878862591649677 ) ) ;
#17589=CARTESIAN_POINT ( 'NONE',  ( 71.02242295334774269, -99.02728775972636299, -55.91838671430374319 ) ) ;
#17607=CARTESIAN_POINT ( 'NONE',  ( 72.54180985774836188, -57.87148204839928667, -35.62222722694667709 ) ) ;
#17615=ORIENTED_EDGE ( 'NONE', *, *, #11679, .F. ) ;
#17650=AXIS2_PLACEMENT_3D ( 'NONE', #40425, #19662, #41560 ) ;
#17664=CONICAL_SURFACE ( 'NONE', #32930, 2.999999999999999556, 0.9599310885968830309 ) ;
#17690=CYLINDRICAL_SURFACE ( 'NONE', #36397, 3.000000000000001776 ) ;
#17695=DIRECTION ( 'NONE',  ( 0.9609149988134843001, -0.1028163501681632064, 0.2570431154366505933 ) ) ;
#17704=ORIENTED_EDGE ( 'NONE', *, *, #37137, .F. ) ;
#17714=CIRCLE ( 'NONE', #29363, 2.999999999999999556 ) ;
#17717=DIRECTION ( 'NONE',  ( 0.7202110682883375858, 0.2576522076061144029, -0.6441361323747234469 ) ) ;
#17748=DIRECTION ( 'NONE',  ( 0.9609149988134837450, -0.1028163501681639419, 0.2570431154366518145 ) ) ;
#17762=EDGE_CURVE ( 'NONE', #23958, #34887, #14081, .T. ) ;
#17764=DIRECTION ( 'NONE',  ( 0.9609149988134837450, -0.1028163501681639419, 0.2570431154366518145 ) ) ;
#17771=CARTESIAN_POINT ( 'NONE',  ( 67.30914723170953096, -55.09414448979863010, -36.13498279219247422 ) ) ;
#17774=CLOSED_SHELL ( 'NONE', ( #19760, #20748, #1365, #11142, #19718, #39380, #35126, #5782, #18026, #36132, #8617, #16853, #31538, #23199, #24289, #13707, #25285, #39956, #3855, #19600, #16713, #1065, #36751, #43152, #38639, #11359, #35324, #32251, #43415, #38918, #1899, #20051, #23856, #38663, #35323, #24491, #4105, #38729, #15016, #27834, #24194, #31145, #17355, #35897, #30354, #39223, #32308, #11556, #7746, #25874, #8940, #19996, #6232, #39519, #41555, #24649, #4717, #38774, #14429, #18905, #29455, #5625, #43816, #21418, #19539, #18676, #16585, #37587, #32249, #39263, #6080, #21769, #23631, #30560, #43180, #16415, #33155, #29527, #24101, #9185, #29848, #9828, #12818, #37294, #3810, #43726, #31054, #28943, #12358, #19985, #30363, #36718, #11420, #22896, #22505, #33630, #10616, #41246, #4087, #10657, #10458, #8383, #38120, #40137, #38126 ) ) ;
#17821=DIRECTION ( 'NONE',  ( 0.9609149988134843001, -0.1028163501681632064, 0.2570431154366505933 ) ) ;
#17829=DIRECTION ( 'NONE',  ( -0.2768435750659239414, -0.3568721902840664151, 0.8921882507333142032 ) ) ;
#17855=EDGE_CURVE ( 'NONE', #15244, #32861, #17714, .T. ) ;
#17877=ORIENTED_EDGE ( 'NONE', *, *, #40253, .F. ) ;
#17911=CARTESIAN_POINT ( 'NONE',  ( 67.30914723170953096, -53.23718887596189120, -35.39220701967414584 ) ) ;
#17913=CARTESIAN_POINT ( 'NONE',  ( 70.19189222814998175, -100.0979043305785581, -53.24182196210380624 ) ) ;
#17915=CIRCLE ( 'NONE', #28146, 2.999999999999999556 ) ;
#17963=AXIS2_PLACEMENT_3D ( 'NONE', #43320, #12089, #8659 ) ;
#17973=DIRECTION ( 'NONE',  ( 0.7871354856660198740, 0.4483307682966886643, 0.4235767337848242442 ) ) ;
#17996=MECHANICAL_DESIGN_GEOMETRIC_PRESENTATION_REPRESENTATION('',(#19467),#4159);
#17997=DIRECTION ( 'NONE',  ( 0.000000000000000000, 0.9284778069183718952, 0.3713878862591649677 ) ) ;
#18012=AXIS2_PLACEMENT_3D ( 'NONE', #33156, #40250, #9017 ) ;
#18015=ORIENTED_EDGE ( 'NONE', *, *, #15886, .T. ) ;
#18026=ADVANCED_FACE ( 'NONE', ( #5944 ), #4119, .T. ) ;
#18029=FACE_OUTER_BOUND ( 'NONE', #16363, .T. ) ;
#18035=CARTESIAN_POINT ( 'NONE',  ( 70.19189222814998175, -59.11650476797663600, -36.84940499091918298 ) ) ;
#18060=ORIENTED_EDGE ( 'NONE', *, *, #40755, .T. ) ;
#18061=CARTESIAN_POINT ( 'NONE',  ( 70.19189222814998175, -52.61716011954800365, -34.24968978710501943 ) ) ;
#18070=CARTESIAN_POINT ( 'NONE',  ( 67.30914723170953096, -60.66501133130886814, -38.36331010974746647 ) ) ;
#18072=ORIENTED_EDGE ( 'NONE', *, *, #8181, .T. ) ;
#18078=VERTEX_POINT ( 'NONE', #28537 ) ;
#18097=DIRECTION ( 'NONE',  ( 0.7871354856660167654, -0.6167752151498625546, -0.002461946824136807422 ) ) ;
#18102=DIRECTION ( 'NONE',  ( -0.000000000000000000, -0.9284778069183721172, -0.3713878862591650232 ) ) ;
#18123=ORIENTED_EDGE ( 'NONE', *, *, #22814, .F. ) ;
#18179=AXIS2_PLACEMENT_3D ( 'NONE', #35291, #652, #21185 ) ;
#18190=ORIENTED_EDGE ( 'NONE', *, *, #42098, .T. ) ;
#18195=DIRECTION ( 'NONE',  ( 0.000000000000000000, 0.9284778069183720062, 0.3713878862591650232 ) ) ;
#18200=CIRCLE ( 'NONE', #19666, 2.999999999999999556 ) ;
#18206=DIRECTION ( 'NONE',  ( 0.9609149988134837450, -0.1028163501681639419, 0.2570431154366518145 ) ) ;
#18221=COLOUR_RGB ( '',0.7921568627450980005, 0.8196078431372548767, 0.9333333333333333481 ) ;
#18252=AXIS2_PLACEMENT_3D ( 'NONE', #8134, #22035, #29097 ) ;
#18276=DIRECTION ( 'NONE',  ( 0.9609149988134837450, -0.1028163501681639419, 0.2570431154366518145 ) ) ;
#18277=DIRECTION ( 'NONE',  ( 0.9609149988134837450, -0.1028163501681639419, 0.2570431154366518145 ) ) ;
#18303=CIRCLE ( 'NONE', #23423, 2.999999999999999556 ) ;
#18314=AXIS2_PLACEMENT_3D ( 'NONE', #27655, #10329, #16265 ) ;
#18335=CARTESIAN_POINT ( 'NONE',  ( 70.19189222814998175, -54.83461124330791847, -35.13666250696951465 ) ) ;
#18338=DIRECTION ( 'NONE',  ( -0.7871354856660202071, 0.6167752151498580027, 0.002461946824133919541 ) ) ;
#18351=ORIENTED_EDGE ( 'NONE', *, *, #34569, .F. ) ;
#18381=DIRECTION ( 'NONE',  ( 0.9705985873829334754, 0.08939452397200674250, -0.2234882575306194330 ) ) ;
#18421=VERTEX_POINT ( 'NONE', #4419 ) ;
#18469=ORIENTED_EDGE ( 'NONE', *, *, #29924, .F. ) ;
#18481=VERTEX_POINT ( 'NONE', #8972 ) ;
#18485=LINE ( 'NONE', #4333, #33078 ) ;
#18495=VECTOR ( 'NONE', #26504, 1000.000000000000227 ) ;
#18505=CARTESIAN_POINT ( 'NONE',  ( 70.19189222814998175, -53.54563792646638376, -34.62107767336419073 ) ) ;
#18517=CARTESIAN_POINT ( 'NONE',  ( 69.36136150295220659, -61.83659016559353461, -34.83262201967072258 ) ) ;
#18545=VERTEX_POINT ( 'NONE', #2568 ) ;
#18597=EDGE_CURVE ( 'NONE', #2964, #23812, #15587, .T. ) ;
#18598=CARTESIAN_POINT ( 'NONE',  ( 67.84197459855160162, -56.44012947280842241, -36.50803721828817316 ) ) ;
#18604=CARTESIAN_POINT ( 'NONE',  ( 70.19189222814998175, -55.19510675323109439, -35.28085945431567438 ) ) ;
#18616=DIRECTION ( 'NONE',  ( 0.9609149988134838560, -0.1028163501681645386, 0.2570431154366520921 ) ) ;
#18629=ORIENTED_EDGE ( 'NONE', *, *, #20936, .T. ) ;
#18647=DIRECTION ( 'NONE',  ( -0.000000000000000000, -0.9284778069183721172, -0.3713878862591650232 ) ) ;
#18649=DIRECTION ( 'NONE',  ( -0.000000000000000000, -0.9284778069183718952, -0.3713878862591649677 ) ) ;
#18653=VECTOR ( 'NONE', #25308, 999.9999999999998863 ) ;
#18676=ADVANCED_FACE ( 'NONE', ( #41792 ), #1720, .T. ) ;
#18679=CIRCLE ( 'NONE', #44177, 4.699999999999999289 ) ;
#18701=CONICAL_SURFACE ( 'NONE', #28896, 2.999999999999999556, 0.9599310885968830309 ) ;
#18734=EDGE_LOOP ( 'NONE', ( #26412, #27883, #19705 ) ) ;
#18739=EDGE_CURVE ( 'NONE', #29216, #37171, #167, .T. ) ;
#18748=EDGE_LOOP ( 'NONE', ( #15474, #5038 ) ) ;
#18754=EDGE_LOOP ( 'NONE', ( #43981, #37874, #26009, #9388, #31433 ) ) ;
#18760=ORIENTED_EDGE ( 'NONE', *, *, #20644, .T. ) ;
#18777=VERTEX_POINT ( 'NONE', #24017 ) ;
#18787=DIRECTION ( 'NONE',  ( -0.000000000000000000, -0.9284778069183721172, -0.3713878862591650232 ) ) ;
#18806=FACE_OUTER_BOUND ( 'NONE', #44789, .T. ) ;
#18823=DIRECTION ( 'NONE',  ( -0.1957579692570466934, -0.9088796992199469349, 0.3682614693641134140 ) ) ;
#18833=CARTESIAN_POINT ( 'NONE',  ( 72.54180985774836188, -51.37213739997068984, -33.02251202313252065 ) ) ;
#18834=LINE ( 'NONE', #4696, #41583 ) ;
#18841=DIRECTION ( 'NONE',  ( -0.000000000000000000, -0.9284778069183720062, -0.3713878862591650232 ) ) ;
#18844=LINE ( 'NONE', #43018, #33744 ) ;
#18853=CIRCLE ( 'NONE', #34873, 2.999999999999999556 ) ;
#18879=ORIENTED_EDGE ( 'NONE', *, *, #44579, .F. ) ;
#18905=ADVANCED_FACE ( 'NONE', ( #25573, #4134 ), #38556, .T. ) ;
#18912=EDGE_CURVE ( 'NONE', #42996, #2964, #38114, .T. ) ;
#18918=CARTESIAN_POINT ( 'NONE',  ( 68.07789357685331311, -68.58957386525776201, -38.44539312525987640 ) ) ;
#18951=DIRECTION ( 'NONE',  ( -0.7871354856660202071, 0.6167752151498580027, 0.002461946824133919541 ) ) ;
#18973=ORIENTED_EDGE ( 'NONE', *, *, #39430, .T. ) ;
#19004=ORIENTED_EDGE ( 'NONE', *, *, #23925, .T. ) ;
#19011=DIRECTION ( 'NONE',  ( -0.9609149988134837450, 0.1028163501681639419, -0.2570431154366518145 ) ) ;
#19015=ORIENTED_EDGE ( 'NONE', *, *, #41411, .T. ) ;
#19038=ORIENTED_EDGE ( 'NONE', *, *, #20015, .T. ) ;
#19056=DIRECTION ( 'NONE',  ( -0.000000000000000000, -0.9284778069183720062, -0.3713878862591650232 ) ) ;
#19059=DIRECTION ( 'NONE',  ( 0.9609149988134843001, -0.1028163501681632064, 0.2570431154366505933 ) ) ;
#19060=CARTESIAN_POINT ( 'NONE',  ( 71.09163384711422395, -63.88803250098678888, -42.12154107070359288 ) ) ;
#19070=LINE ( 'NONE', #8807, #4616 ) ;
#19087=FACE_OUTER_BOUND ( 'NONE', #9236, .T. ) ;
#19123=DIRECTION ( 'NONE',  ( -0.000000000000000000, -0.9284778069183721172, -0.3713878862591650232 ) ) ;
#19126=AXIS2_PLACEMENT_3D ( 'NONE', #22556, #29177, #4999 ) ;
#19153=AXIS2_PLACEMENT_3D ( 'NONE', #38637, #8102, #28852 ) ;
#19163=VERTEX_POINT ( 'NONE', #18517 ) ;
#19172=CARTESIAN_POINT ( 'NONE',  ( 70.89562859596755118, -66.92613143246303764, -42.60403544796190545 ) ) ;
#19180=DIRECTION ( 'NONE',  ( -0.2768435750659266059, -0.3568721902840680249, 0.8921882507333128709 ) ) ;
#19191=ORIENTED_EDGE ( 'NONE', *, *, #30164, .T. ) ;
#19204=ORIENTED_EDGE ( 'NONE', *, *, #9220, .T. ) ;
#19223=AXIS2_PLACEMENT_3D ( 'NONE', #16991, #37250, #33372 ) ;
#19251=EDGE_CURVE ( 'NONE', #27626, #25810, #9152, .T. ) ;
#19270=DIRECTION ( 'NONE',  ( 0.9609149988134843001, -0.1028163501681632064, 0.2570431154366505933 ) ) ;
#19301=CARTESIAN_POINT ( 'NONE',  ( 73.07463722459043254, -52.92560917005250332, -33.47856044079506432 ) ) ;
#19302=ORIENTED_EDGE ( 'NONE', *, *, #4309, .F. ) ;
#19317=CARTESIAN_POINT ( 'NONE',  ( 73.07463722459043254, -60.14594483832745198, -36.36666953930154023 ) ) ;
#19350=CARTESIAN_POINT ( 'NONE',  ( 70.19189222814998175, -67.83330054016514055, -40.33609291459782753 ) ) ;
#19357=CARTESIAN_POINT ( 'NONE',  ( 70.19189222814998175, -59.11650476797663600, -36.84940499091918298 ) ) ;
#19371=CARTESIAN_POINT ( 'NONE',  ( 70.19189222814998175, -52.61716011954800365, -34.24968978710501943 ) ) ;
#19375=CARTESIAN_POINT ( 'NONE',  ( 70.19189222814998175, -54.47411573338475677, -34.99246555962335492 ) ) ;
#19385=ORIENTED_EDGE ( 'NONE', *, *, #25570, .T. ) ;
#19390=DIRECTION ( 'NONE',  ( 0.000000000000000000, 0.9284778069183720062, 0.3713878862591650232 ) ) ;
#19395=CARTESIAN_POINT ( 'NONE',  ( 70.19189222814998175, -57.25954915413987578, -36.10662921840084749 ) ) ;
#19402=ORIENTED_EDGE ( 'NONE', *, *, #23992, .T. ) ;
#19416=ORIENTED_EDGE ( 'NONE', *, *, #11637, .T. ) ;
#19437=EDGE_CURVE ( 'NONE', #11292, #34097, #29443, .T. ) ;
#19467=STYLED_ITEM('',(#45190),#6206);
#19473=EDGE_LOOP ( 'NONE', ( #964, #27553, #43561, #14093, #12741, #20082 ) ) ;
#19495=VECTOR ( 'NONE', #16085, 1000.000000000000000 ) ;
#19524=VERTEX_POINT ( 'NONE', #7075 ) ;
#19539=ADVANCED_FACE ( 'NONE', ( #6633 ), #6016, .F. ) ;
#19573=CYLINDRICAL_SURFACE ( 'NONE', #27564, 3.000000000000001776 ) ;
#19580=DIRECTION ( 'NONE',  ( -0.9609149988134837450, 0.1028163501681639419, -0.2570431154366518145 ) ) ;
#19600=ADVANCED_FACE ( 'NONE', ( #10 ), #6759, .T. ) ;
#19624=DIRECTION ( 'NONE',  ( -0.000000000000000000, -0.9284778069183720062, -0.3713878862591650232 ) ) ;
#19653=FACE_OUTER_BOUND ( 'NONE', #5167, .T. ) ;
#19662=DIRECTION ( 'NONE',  ( -0.000000000000000000, -0.9284778069183721172, -0.3713878862591650232 ) ) ;
#19666=AXIS2_PLACEMENT_3D ( 'NONE', #28487, #10488, #28038 ) ;
#19668=ORIENTED_EDGE ( 'NONE', *, *, #17337, .T. ) ;
#19681=DIRECTION ( 'NONE',  ( -0.000000000000000000, -0.9284778069183718952, -0.3713878862591649677 ) ) ;
#19685=CIRCLE ( 'NONE', #27, 2.999999999999999556 ) ;
#19705=ORIENTED_EDGE ( 'NONE', *, *, #19251, .T. ) ;
#19710=CIRCLE ( 'NONE', #18252, 2.999999999999999556 ) ;
#19718=ADVANCED_FACE ( 'NONE', ( #13484 ), #9679, .T. ) ;
#19746=ORIENTED_EDGE ( 'NONE', *, *, #587, .F. ) ;
#19760=ADVANCED_FACE ( 'NONE', ( #15258 ), #28505, .T. ) ;
#19764=DIRECTION ( 'NONE',  ( -0.000000000000000000, -0.9284778069183721172, -0.3713878862591650232 ) ) ;
#19781=ORIENTED_EDGE ( 'NONE', *, *, #4309, .T. ) ;
#19809=FACE_OUTER_BOUND ( 'NONE', #20616, .T. ) ;
#19823=VERTEX_POINT ( 'NONE', #16393 ) ;
#19833=CONICAL_SURFACE ( 'NONE', #3104, 2.445500000000004448, 0.9599310885968757034 ) ;
#19859=ORIENTED_EDGE ( 'NONE', *, *, #30017, .T. ) ;
#19893=DIRECTION ( 'NONE',  ( 0.9609149988134837450, -0.1028163501681639419, 0.2570431154366518145 ) ) ;
#19894=VERTEX_POINT ( 'NONE', #8421 ) ;
#19913=CARTESIAN_POINT ( 'NONE',  ( 68.07789357685331311, -68.58957386525776201, -38.44539312525988350 ) ) ;
#19914=LINE ( 'NONE', #3250, #10984 ) ;
#19925=ORIENTED_EDGE ( 'NONE', *, *, #796, .F. ) ;
#19931=ORIENTED_EDGE ( 'NONE', *, *, #34052, .T. ) ;
#19932=DIRECTION ( 'NONE',  ( 0.000000000000000000, 0.9284778069183720062, 0.3713878862591650232 ) ) ;
#19940=DIRECTION ( 'NONE',  ( -0.9609149988134837450, 0.1028163501681639419, -0.2570431154366518145 ) ) ;
#19956=ORIENTED_EDGE ( 'NONE', *, *, #33402, .T. ) ;
#19962=CIRCLE ( 'NONE', #11240, 2.999999999999999556 ) ;
#19966=LINE ( 'NONE', #41180, #33998 ) ;
#19969=LINE ( 'NONE', #13807, #25543 ) ;
#19985=ADVANCED_FACE ( 'NONE', ( #19809 ), #191, .T. ) ;
#19994=AXIS2_PLACEMENT_3D ( 'NONE', #34827, #44915, #10034 ) ;
#19996=ADVANCED_FACE ( 'NONE', ( #36891 ), #40333, .T. ) ;
#19998=CARTESIAN_POINT ( 'NONE',  ( 70.19189222814998175, -58.54852247098141049, -36.62221405200617141 ) ) ;
#20003=DIRECTION ( 'NONE',  ( 0.9609149988134843001, -0.1028163501681632064, 0.2570431154366505933 ) ) ;
#20010=ORIENTED_EDGE ( 'NONE', *, *, #33178, .F. ) ;
#20015=EDGE_CURVE ( 'NONE', #2361, #42481, #9098, .T. ) ;
#20033=ORIENTED_EDGE ( 'NONE', *, *, #19437, .T. ) ;
#20041=FILL_AREA_STYLE ('',( #37350 ) ) ;
#20051=ADVANCED_FACE ( 'NONE', ( #8868 ), #11116, .T. ) ;
#20056=AXIS2_PLACEMENT_3D ( 'NONE', #20344, #2999, #16924 ) ;
#20061=DIRECTION ( 'NONE',  ( -0.000000000000000000, -0.9284778069183721172, -0.3713878862591650232 ) ) ;
#20082=ORIENTED_EDGE ( 'NONE', *, *, #12252, .F. ) ;
#20102=AXIS2_PLACEMENT_3D ( 'NONE', #3056, #16984, #30876 ) ;
#20113=VERTEX_POINT ( 'NONE', #37115 ) ;
#20119=VERTEX_POINT ( 'NONE', #24139 ) ;
#20140=EDGE_LOOP ( 'NONE', ( #30925, #32470, #13192, #18760, #33088 ) ) ;
#20144=EDGE_CURVE ( 'NONE', #25485, #33632, #14067, .T. ) ;
#20150=ORIENTED_EDGE ( 'NONE', *, *, #5262, .T. ) ;
#20162=VECTOR ( 'NONE', #33427, 1000.000000000000227 ) ;
#20188=DIRECTION ( 'NONE',  ( -0.000000000000000000, -0.9284778069183718952, -0.3713878862591649677 ) ) ;
#20227=DIRECTION ( 'NONE',  ( -0.2768435750659241079, -0.3568721902840695792, 0.8921882507333129819 ) ) ;
#20236=DIRECTION ( 'NONE',  ( 0.7871354856660198740, 0.4483307682966886643, 0.4235767337848242442 ) ) ;
#20238=VECTOR ( 'NONE', #27004, 1000.000000000000227 ) ;
#20242=ORIENTED_EDGE ( 'NONE', *, *, #7655, .T. ) ;
#20255=ORIENTED_EDGE ( 'NONE', *, *, #20644, .F. ) ;
#20256=CARTESIAN_POINT ( 'NONE',  ( 67.37136766119182596, -70.31694239570130378, -42.20474206142759499 ) ) ;
#20264=ORIENTED_EDGE ( 'NONE', *, *, #3550, .F. ) ;
#20278=CARTESIAN_POINT ( 'NONE',  ( 67.84197459855160162, -51.79774043821656448, -34.65109778699235221 ) ) ;
#20280=ORIENTED_EDGE ( 'NONE', *, *, #44070, .T. ) ;
#20297=ORIENTED_EDGE ( 'NONE', *, *, #5784, .T. ) ;
#20329=VERTEX_POINT ( 'NONE', #44441 ) ;
#20338=ORIENTED_EDGE ( 'NONE', *, *, #37271, .F. ) ;
#20344=CARTESIAN_POINT ( 'NONE',  ( 70.19189222814998175, -54.26662894631272849, -34.90947156805651019 ) ) ;
#20345=DIRECTION ( 'NONE',  ( 0.9609149988134837450, -0.1028163501681639419, 0.2570431154366518145 ) ) ;
#20389=AXIS2_PLACEMENT_3D ( 'NONE', #19998, #37538, #13393 ) ;
#20409=CARTESIAN_POINT ( 'NONE',  ( 73.07463722459043254, -51.78964457606210203, -33.02417856296905541 ) ) ;
#20449=DIRECTION ( 'NONE',  ( 0.000000000000000000, 0.9284778069183718952, 0.3713878862591649677 ) ) ;
#20451=ORIENTED_EDGE ( 'NONE', *, *, #30928, .F. ) ;
#20465=CARTESIAN_POINT ( 'NONE',  ( 70.19189222814998175, -61.69445140165969121, -37.88057465812982372 ) ) ;
#20467=ORIENTED_EDGE ( 'NONE', *, *, #23236, .F. ) ;
#20470=FACE_OUTER_BOUND ( 'NONE', #18734, .T. ) ;
#20489=ORIENTED_EDGE ( 'NONE', *, *, #15751, .T. ) ;
#20499=AXIS2_PLACEMENT_3D ( 'NONE', #9683, #16759, #9918 ) ;
#20508=CONICAL_SURFACE ( 'NONE', #26321, 2.541999999999999371, 1.047197551196596299 ) ;
#20510=DIRECTION ( 'NONE',  ( -0.000000000000000000, -0.9284778069183718952, -0.3713878862591649677 ) ) ;
#20516=CARTESIAN_POINT ( 'NONE',  ( 71.02242295334774269, -61.55231263772585493, -40.92852729658892486 ) ) ;
#20545=DIRECTION ( 'NONE',  ( 0.000000000000000000, 0.9284778069183720062, 0.3713878862591650232 ) ) ;
#20558=EDGE_CURVE ( 'NONE', #33021, #29611, #8960, .T. ) ;
#20574=CARTESIAN_POINT ( 'NONE',  ( 69.36136150295220659, -57.19420113100166958, -32.97568258837489452 ) ) ;
#20595=AXIS2_PLACEMENT_3D ( 'NONE', #28949, #42857, #42187 ) ;
#20598=ORIENTED_EDGE ( 'NONE', *, *, #41658, .T. ) ;
#20614=VERTEX_POINT ( 'NONE', #40842 ) ;
#20616=EDGE_LOOP ( 'NONE', ( #1435, #6239, #12068, #24613, #41995 ) ) ;
#20640=ORIENTED_EDGE ( 'NONE', *, *, #40516, .T. ) ;
#20644=EDGE_CURVE ( 'NONE', #5080, #38926, #10432, .T. ) ;
#20657=DIRECTION ( 'NONE',  ( -0.000000000000000000, -0.9284778069183721172, -0.3713878862591650232 ) ) ;
#20658=EDGE_CURVE ( 'NONE', #27773, #27364, #12346, .T. ) ;
#20711=ORIENTED_EDGE ( 'NONE', *, *, #3022, .F. ) ;
#20748=ADVANCED_FACE ( 'NONE', ( #5264 ), #16983, .T. ) ;
#20754=DIRECTION ( 'NONE',  ( -0.000000000000000000, -0.9284778069183721172, -0.3713878862591650232 ) ) ;
#20777=AXIS2_PLACEMENT_3D ( 'NONE', #36056, #8482, #1624 ) ;
#20785=CARTESIAN_POINT ( 'NONE',  ( 67.30914723170953096, -56.02262229671700311, -36.50637067845163841 ) ) ;
#20787=LINE ( 'NONE', #27636, #38602 ) ;
#20801=DIRECTION ( 'NONE',  ( -0.000000000000000000, -0.9284778069183721172, -0.3713878862591650232 ) ) ;
#20803=VERTEX_POINT ( 'NONE', #13023 ) ;
#20814=ORIENTED_EDGE ( 'NONE', *, *, #31182, .T. ) ;
#20838=FACE_OUTER_BOUND ( 'NONE', #3277, .T. ) ;
#20841=VECTOR ( 'NONE', #12377, 1000.000000000000227 ) ;
#20842=CARTESIAN_POINT ( 'NONE',  ( 70.19189222814998175, -100.0979043305785581, -53.24182196210380624 ) ) ;
#20845=DIRECTION ( 'NONE',  ( -0.7871354856660162103, -0.4483307682966942709, -0.4235767337848251879 ) ) ;
#20893=EDGE_CURVE ( 'NONE', #25485, #39549, #13697, .T. ) ;
#20894=DIRECTION ( 'NONE',  ( -0.000000000000000000, -0.9284778069183721172, -0.3713878862591650232 ) ) ;
#20907=DIRECTION ( 'NONE',  ( -0.2768435750659239414, -0.3568721902840664151, 0.8921882507333142032 ) ) ;
#20929=EDGE_LOOP ( 'NONE', ( #19746, #4255, #45101, #25507, #26606 ) ) ;
#20936=EDGE_CURVE ( 'NONE', #3470, #14232, #2, .T. ) ;
#20949=CIRCLE ( 'NONE', #10764, 2.999999999999999556 ) ;
#20957=FACE_OUTER_BOUND ( 'NONE', #12575, .T. ) ;
#20983=CARTESIAN_POINT ( 'NONE',  ( 70.19189222814998175, -57.25954915413987578, -36.10662921840084749 ) ) ;
#20985=DIRECTION ( 'NONE',  ( -0.000000000000000000, -0.9284778069183720062, -0.3713878862591650232 ) ) ;
#20997=ORIENTED_EDGE ( 'NONE', *, *, #935, .F. ) ;
#21005=AXIS2_PLACEMENT_3D ( 'NONE', #19350, #19123, #8858 ) ;
#21018=EDGE_CURVE ( 'NONE', #5955, #9699, #19070, .T. ) ;
#21021=ORIENTED_EDGE ( 'NONE', *, *, #179, .F. ) ;
#21045=VERTEX_POINT ( 'NONE', #5384 ) ;
#21046=DIRECTION ( 'NONE',  ( -0.9609149988134837450, 0.1028163501681639419, -0.2570431154366518145 ) ) ;
#21066=AXIS2_PLACEMENT_3D ( 'NONE', #15885, #29781, #32737 ) ;
#21087=EDGE_CURVE ( 'NONE', #31092, #43396, #29334, .T. ) ;
#21097=VECTOR ( 'NONE', #35113, 1000.000000000000114 ) ;
#21106=CONICAL_SURFACE ( 'NONE', #20389, 2.445500000000004448, 0.9599310885968757034 ) ;
#21161=ORIENTED_EDGE ( 'NONE', *, *, #6632, .T. ) ;
#21181=ORIENTED_EDGE ( 'NONE', *, *, #27844, .F. ) ;
#21185=DIRECTION ( 'NONE',  ( -0.9609149988134837450, 0.1028163501681639419, -0.2570431154366518145 ) ) ;
#21202=DIRECTION ( 'NONE',  ( -0.9609149988134837450, 0.1028163501681639419, -0.2570431154366518145 ) ) ;
#21211=AXIS2_PLACEMENT_3D ( 'NONE', #23668, #37323, #41673 ) ;
#21214=VERTEX_POINT ( 'NONE', #8362 ) ;
#21255=ORIENTED_EDGE ( 'NONE', *, *, #28168, .F. ) ;
#21289=FACE_OUTER_BOUND ( 'NONE', #2074, .T. ) ;
#21309=EDGE_CURVE ( 'NONE', #32855, #20113, #18844, .T. ) ;
#21318=ORIENTED_EDGE ( 'NONE', *, *, #34504, .T. ) ;
#21326=CIRCLE ( 'NONE', #14784, 2.541999999999999371 ) ;
#21356=VECTOR ( 'NONE', #38023, 1000.000000000000227 ) ;
#21379=ORIENTED_EDGE ( 'NONE', *, *, #36438, .F. ) ;
#21384=ORIENTED_EDGE ( 'NONE', *, *, #44070, .F. ) ;
#21395=FACE_OUTER_BOUND ( 'NONE', #18748, .T. ) ;
#21408=DIRECTION ( 'NONE',  ( -0.000000000000000000, -0.9284778069183721172, -0.3713878862591650232 ) ) ;
#21409=DIRECTION ( 'NONE',  ( -0.000000000000000000, -0.9284778069183721172, -0.3713878862591650232 ) ) ;
#21418=ADVANCED_FACE ( 'NONE', ( #35545 ), #8995, .T. ) ;
#21450=VECTOR ( 'NONE', #37881, 1000.000000000000227 ) ;
#21487=ORIENTED_EDGE ( 'NONE', *, *, #41286, .T. ) ;
#21490=LINE ( 'NONE', #42696, #38240 ) ;
#21514=VECTOR ( 'NONE', #14005, 1000.000000000000227 ) ;
#21544=LINE ( 'NONE', #7630, #26183 ) ;
#21606=CARTESIAN_POINT ( 'NONE',  ( 67.30914723170953096, -53.23718887596189120, -35.39220701967414584 ) ) ;
#21622=CIRCLE ( 'NONE', #37676, 2.999999999999999556 ) ;
#21629=ORIENTED_EDGE ( 'NONE', *, *, #20658, .T. ) ;
#21638=FACE_OUTER_BOUND ( 'NONE', #42147, .T. ) ;
#21649=DIRECTION ( 'NONE',  ( 0.000000000000000000, 0.000000000000000000, 1.000000000000000000 ) ) ;
#21695=EDGE_LOOP ( 'NONE', ( #29239, #42967, #43508, #8259, #11467 ) ) ;
#21707=CARTESIAN_POINT ( 'NONE',  ( 67.84197459855160162, -50.86926263129819148, -34.27970990073318802 ) ) ;
#21716=EDGE_CURVE ( 'NONE', #22284, #20119, #2475, .T. ) ;
#21755=EDGE_CURVE ( 'NONE', #44682, #25810, #43210, .T. ) ;
#21769=ADVANCED_FACE ( 'NONE', ( #22774 ), #32998, .T. ) ;
#21775=ORIENTED_EDGE ( 'NONE', *, *, #27880, .F. ) ;
#21845=CIRCLE ( 'NONE', #23319, 2.999999999999999556 ) ;
#21856=DIRECTION ( 'NONE',  ( 0.9609149988134837450, -0.1028163501681639419, 0.2570431154366518145 ) ) ;
#21858=CIRCLE ( 'NONE', #3660, 3.249999999999996003 ) ;
#21859=DIRECTION ( 'NONE',  ( 0.9609149988134837450, -0.1028163501681639419, 0.2570431154366518145 ) ) ;
#21860=CARTESIAN_POINT ( 'NONE',  ( 73.07463722459043254, -56.63952039772598823, -34.96411198583172819 ) ) ;
#21862=CIRCLE ( 'NONE', #22610, 2.999999999999999556 ) ;
#21879=CARTESIAN_POINT ( 'NONE',  ( 67.30914723170953096, -59.73653352439050934, -37.99192222348830938 ) ) ;
#21894=FACE_OUTER_BOUND ( 'NONE', #28313, .T. ) ;
#21911=CONICAL_SURFACE ( 'NONE', #12456, 2.445500000000004448, 0.9599310885968757034 ) ;
#21946=CIRCLE ( 'NONE', #33581, 2.999999999999999556 ) ;
#21955=CIRCLE ( 'NONE', #5218, 2.999999999999999556 ) ;
#21961=DIRECTION ( 'NONE',  ( -0.000000000000000000, -0.9284778069183721172, -0.3713878862591650232 ) ) ;
#21967=DIRECTION ( 'NONE',  ( -0.000000000000000000, -0.9284778069183721172, -0.3713878862591650232 ) ) ;
#21972=CARTESIAN_POINT ( 'NONE',  ( 70.19189222814998175, -62.62292920857806422, -38.25196254438899501 ) ) ;
#22035=DIRECTION ( 'NONE',  ( -0.000000000000000000, -0.9284778069183721172, -0.3713878862591650232 ) ) ;
#22042=DIRECTION ( 'NONE',  ( 0.9609149988134843001, -0.1028163501681632064, 0.2570431154366505933 ) ) ;
#22046=ORIENTED_EDGE ( 'NONE', *, *, #6157, .F. ) ;
#22055=CIRCLE ( 'NONE', #38807, 2.999999999999999556 ) ;
#22085=EDGE_LOOP ( 'NONE', ( #22417, #24803, #26269 ) ) ;
#22093=EDGE_LOOP ( 'NONE', ( #27102, #9495, #16052, #41426, #11895 ) ) ;
#22114=DIRECTION ( 'NONE',  ( -0.000000000000000000, -0.9284778069183721172, -0.3713878862591650232 ) ) ;
#22125=DIRECTION ( 'NONE',  ( -0.000000000000000000, -0.9284778069183718952, -0.3713878862591649677 ) ) ;
#22169=VERTEX_POINT ( 'NONE', #21606 ) ;
#22170=ORIENTED_EDGE ( 'NONE', *, *, #24486, .T. ) ;
#22192=ORIENTED_EDGE ( 'NONE', *, *, #26163, .T. ) ;
#22199=CIRCLE ( 'NONE', #22912, 2.445500000000004448 ) ;
#22201=FACE_OUTER_BOUND ( 'NONE', #34473, .T. ) ;
#22212=ORIENTED_EDGE ( 'NONE', *, *, #8181, .F. ) ;
#22225=LINE ( 'NONE', #17911, #37346 ) ;
#22226=LINE ( 'NONE', #40003, #7706 ) ;
#22236=EDGE_CURVE ( 'NONE', #29748, #44499, #35901, .T. ) ;
#22250=EDGE_CURVE ( 'NONE', #20329, #34274, #40287, .T. ) ;
#22257=CARTESIAN_POINT ( 'NONE',  ( 68.89072742534011695, -72.01748991317985826, -37.14555542905099372 ) ) ;
#22267=ORIENTED_EDGE ( 'NONE', *, *, #40464, .F. ) ;
#22269=CONICAL_SURFACE ( 'NONE', #42680, 2.445500000000004448, 0.9599310885968757034 ) ;
#22284=VERTEX_POINT ( 'NONE', #7691 ) ;
#22292=CARTESIAN_POINT ( 'NONE',  ( 70.19189222814998175, -100.0979043305785581, -53.24182196210380624 ) ) ;
#22312=CARTESIAN_POINT ( 'NONE',  ( 67.30914723170953096, -50.45175545520677929, -34.27804336089664616 ) ) ;
#22315=ORIENTED_EDGE ( 'NONE', *, *, #14542, .F. ) ;
#22317=CARTESIAN_POINT ( 'NONE',  ( 70.19189222814998175, -60.97346038181336070, -37.59218076343751136 ) ) ;
#22324=DIRECTION ( 'NONE',  ( -0.2407039305251456596, 0.3604685577742790525, -0.9011792478113757054 ) ) ;
#22327=DIRECTION ( 'NONE',  ( 0.000000000000000000, 0.9284778069183720062, 0.3713878862591650232 ) ) ;
#22349=CARTESIAN_POINT ( 'NONE',  ( 70.19189222814998175, -53.90613343638955968, -34.76527462071035046 ) ) ;
#22367=DIRECTION ( 'NONE',  ( 0.000000000000000000, 0.9284778069183720062, 0.3713878862591650232 ) ) ;
#22398=CARTESIAN_POINT ( 'NONE',  ( 67.30914723170953096, -61.59348913822725535, -38.73469799600663777 ) ) ;
#22399=ORIENTED_EDGE ( 'NONE', *, *, #33100, .F. ) ;
#22410=ORIENTED_EDGE ( 'NONE', *, *, #11706, .F. ) ;
#22417=ORIENTED_EDGE ( 'NONE', *, *, #38681, .F. ) ;
#22449=DIRECTION ( 'NONE',  ( -0.000000000000000000, -0.9284778069183721172, -0.3713878862591650232 ) ) ;
#22452=DIRECTION ( 'NONE',  ( -0.000000000000000000, -0.9284778069183721172, -0.3713878862591650232 ) ) ;
#22469=LINE ( 'NONE', #12448, #19495 ) ;
#22475=FACE_OUTER_BOUND ( 'NONE', #40176, .T. ) ;
#22504=CARTESIAN_POINT ( 'NONE',  ( 67.30914723170953096, -53.02970208888985582, -35.30921302810730111 ) ) ;
#22505=ADVANCED_FACE ( 'NONE', ( #40055 ), #12257, .T. ) ;
#22532=CARTESIAN_POINT ( 'NONE',  ( 69.36136150295220659, -101.1685209014307674, -50.56525720990386219 ) ) ;
#22556=CARTESIAN_POINT ( 'NONE',  ( 68.07789357685331311, -68.58957386525776201, -38.44539312525988350 ) ) ;
#22560=AXIS2_PLACEMENT_3D ( 'NONE', #13959, #20801, #487 ) ;
#22570=AXIS2_PLACEMENT_3D ( 'NONE', #22630, #21961, #42497 ) ;
#22578=EDGE_LOOP ( 'NONE', ( #5708, #29007, #14123, #2597, #29451 ) ) ;
#22610=AXIS2_PLACEMENT_3D ( 'NONE', #33092, #2317, #1861 ) ;
#22615=ORIENTED_EDGE ( 'NONE', *, *, #22638, .T. ) ;
#22630=CARTESIAN_POINT ( 'NONE',  ( 70.19189222814998175, -62.62292920857806422, -38.25196254438899501 ) ) ;
#22638=EDGE_CURVE ( 'NONE', #29032, #36176, #41798, .T. ) ;
#22640=ORIENTED_EDGE ( 'NONE', *, *, #18912, .T. ) ;
#22641=CIRCLE ( 'NONE', #32100, 0.3000000000000022093 ) ;
#22656=CARTESIAN_POINT ( 'NONE',  ( 69.36136150295220659, -53.68777669040021294, -31.57312503490508604 ) ) ;
#22709=FACE_OUTER_BOUND ( 'NONE', #37499, .T. ) ;
#22713=DIRECTION ( 'NONE',  ( 0.9609149988134837450, -0.1028163501681639419, 0.2570431154366518145 ) ) ;
#22728=AXIS2_PLACEMENT_3D ( 'NONE', #2553, #32553, #18206 ) ;
#22746=AXIS2_PLACEMENT_3D ( 'NONE', #3205, #38296, #17130 ) ;
#22760=EDGE_CURVE ( 'NONE', #14232, #29216, #6102, .T. ) ;
#22768=DIRECTION ( 'NONE',  ( -0.9609149988134837450, 0.1028163501681639419, -0.2570431154366518145 ) ) ;
#22774=FACE_OUTER_BOUND ( 'NONE', #6186, .T. ) ;
#22804=EDGE_CURVE ( 'NONE', #18421, #41822, #15574, .T. ) ;
#22807=CARTESIAN_POINT ( 'NONE',  ( 70.19189222814998175, -57.25954915413987578, -36.10662921840084749 ) ) ;
#22814=EDGE_CURVE ( 'NONE', #39438, #20119, #43967, .T. ) ;
#22838=EDGE_CURVE ( 'NONE', #10520, #43489, #26491, .T. ) ;
#22852=CARTESIAN_POINT ( 'NONE',  ( 70.19189222814998175, -100.0979043305785581, -53.24182196210380624 ) ) ;
#22862=DIRECTION ( 'NONE',  ( 0.1957579692570465546, -0.4041862076864165543, -0.8934832550128906092 ) ) ;
#22896=ADVANCED_FACE ( 'NONE', ( #5121 ), #1734, .T. ) ;
#22908=VERTEX_POINT ( 'NONE', #15851 ) ;
#22912=AXIS2_PLACEMENT_3D ( 'NONE', #40529, #37314, #20003 ) ;
#22956=CARTESIAN_POINT ( 'NONE',  ( 71.02242295334774269, -60.62383483080748903, -40.55713941032976066 ) ) ;
#22978=VECTOR ( 'NONE', #41591, 1000.000000000000227 ) ;
#22992=ORIENTED_EDGE ( 'NONE', *, *, #43882, .F. ) ;
#23009=CIRCLE ( 'NONE', #32438, 2.999999999999999556 ) ;
#23014=AXIS2_PLACEMENT_3D ( 'NONE', #9897, #10945, #4311 ) ;
#23021=DIRECTION ( 'NONE',  ( 0.9609149988134837450, -0.1028163501681639419, 0.2570431154366518145 ) ) ;
#23080=EDGE_CURVE ( 'NONE', #18545, #20614, #30134, .T. ) ;
#23101=DIRECTION ( 'NONE',  ( -0.000000000000000000, -0.9284778069183721172, -0.3713878862591650232 ) ) ;
#23104=EDGE_CURVE ( 'NONE', #16491, #19163, #13413, .T. ) ;
#23137=EDGE_LOOP ( 'NONE', ( #4768, #3493, #11442, #24687, #43994 ) ) ;
#23146=DIRECTION ( 'NONE',  ( 0.7871354856660198740, 0.4483307682966886643, 0.4235767337848242442 ) ) ;
#23148=CARTESIAN_POINT ( 'NONE',  ( 73.07463722459043254, -61.28190943231786036, -36.82105141712754914 ) ) ;
#23183=EDGE_LOOP ( 'NONE', ( #43639, #23703, #1552 ) ) ;
#23189=DIRECTION ( 'NONE',  ( -0.000000000000000000, -0.9284778069183718952, -0.3713878862591649677 ) ) ;
#23194=DIRECTION ( 'NONE',  ( 0.9609149988134834119, -0.1028163501681648995, 0.2570431154366529802 ) ) ;
#23195=AXIS2_PLACEMENT_3D ( 'NONE', #877, #42167, #14345 ) ;
#23197=CARTESIAN_POINT ( 'NONE',  ( 70.89841814381148311, -68.89136543047671069, -37.69090763720760151 ) ) ;
#23199=ADVANCED_FACE ( 'NONE', ( #27471 ), #3916, .T. ) ;
#23202=DIRECTION ( 'NONE',  ( -0.000000000000000000, -0.9284778069183720062, -0.3713878862591650232 ) ) ;
#23221=ORIENTED_EDGE ( 'NONE', *, *, #37007, .F. ) ;
#23236=EDGE_CURVE ( 'NONE', #42441, #26037, #31986, .T. ) ;
#23245=VERTEX_POINT ( 'NONE', #24053 ) ;
#23258=CIRCLE ( 'NONE', #43634, 2.999999999999999556 ) ;
#23267=CARTESIAN_POINT ( 'NONE',  ( 70.19189222814998175, -50.76020450571126474, -33.50691401458669105 ) ) ;
#23278=ORIENTED_EDGE ( 'NONE', *, *, #32840, .F. ) ;
#23284=DIRECTION ( 'NONE',  ( 0.9609149988134833009, -0.1028163501681649411, 0.2570431154366530913 ) ) ;
#23292=ORIENTED_EDGE ( 'NONE', *, *, #2559, .F. ) ;
#23319=AXIS2_PLACEMENT_3D ( 'NONE', #28711, #7948, #21859 ) ;
#23322=ORIENTED_EDGE ( 'NONE', *, *, #4956, .F. ) ;
#23325=CARTESIAN_POINT ( 'NONE',  ( 70.19189222814998175, -100.0979043305785581, -53.24182196210380624 ) ) ;
#23388=EDGE_CURVE ( 'NONE', #37171, #38683, #10194, .T. ) ;
#23401=ORIENTED_EDGE ( 'NONE', *, *, #33100, .T. ) ;
#23409=ORIENTED_EDGE ( 'NONE', *, *, #28101, .T. ) ;
#23410=VECTOR ( 'NONE', #28287, 999.9999999999998863 ) ;
#23417=DIRECTION ( 'NONE',  ( 0.9609149988134837450, -0.1028163501681639419, 0.2570431154366518145 ) ) ;
#23419=EDGE_CURVE ( 'NONE', #38926, #5080, #32011, .T. ) ;
#23423=AXIS2_PLACEMENT_3D ( 'NONE', #33145, #36123, #15616 ) ;
#23427=DIRECTION ( 'NONE',  ( -0.9609149988134837450, 0.1028163501681639419, -0.2570431154366518145 ) ) ;
#23436=ORIENTED_EDGE ( 'NONE', *, *, #40911, .T. ) ;
#23459=LINE ( 'NONE', #37344, #13172 ) ;
#23460=VERTEX_POINT ( 'NONE', #1210 ) ;
#23464=( LENGTH_UNIT ( ) NAMED_UNIT ( * ) SI_UNIT ( .MILLI., .METRE. ) );
#23472=CARTESIAN_POINT ( 'NONE',  ( 70.19189222814998175, -60.04498257489500190, -37.22079287717834717 ) ) ;
#23480=LINE ( 'NONE', #9800, #9251 ) ;
#23482=DIRECTION ( 'NONE',  ( -0.000000000000000000, -0.9284778069183718952, -0.3713878862591649677 ) ) ;
#23489=VECTOR ( 'NONE', #42219, 1000.000000000000227 ) ;
#23503=FACE_OUTER_BOUND ( 'NONE', #2325, .T. ) ;
#23504=CARTESIAN_POINT ( 'NONE',  ( 70.19189222814998175, -51.12070001563444066, -33.65111096193285078 ) ) ;
#23524=ORIENTED_EDGE ( 'NONE', *, *, #41607, .F. ) ;
#23525=AXIS2_PLACEMENT_3D ( 'NONE', #5213, #43985, #22768 ) ;
#23553=ORIENTED_EDGE ( 'NONE', *, *, #39833, .T. ) ;
#23557=CARTESIAN_POINT ( 'NONE',  ( 69.36136150295220659, -101.1685209014307674, -50.56525720990386219 ) ) ;
#23583=EDGE_LOOP ( 'NONE', ( #43201, #8026, #19956, #1854, #44094 ) ) ;
#23599=AXIS2_PLACEMENT_3D ( 'NONE', #25441, #39343, #35906 ) ;
#23613=ORIENTED_EDGE ( 'NONE', *, *, #8588, .F. ) ;
#23631=ADVANCED_FACE ( 'NONE', ( #25614 ), #9469, .T. ) ;
#23647=EDGE_LOOP ( 'NONE', ( #3295, #25848, #36886, #21318, #38310 ) ) ;
#23668=CARTESIAN_POINT ( 'NONE',  ( 68.07789357685331311, -68.58957386525776201, -38.44539312525988350 ) ) ;
#23682=LINE ( 'NONE', #20256, #25512 ) ;
#23691=CIRCLE ( 'NONE', #3988, 2.999999999999999556 ) ;
#23703=ORIENTED_EDGE ( 'NONE', *, *, #34491, .F. ) ;
#23727=EDGE_CURVE ( 'NONE', #29197, #8760, #37114, .T. ) ;
#23753=AXIS2_PLACEMENT_3D ( 'NONE', #34717, #27008, #82 ) ;
#23763=ORIENTED_EDGE ( 'NONE', *, *, #24486, .F. ) ;
#23778=ORIENTED_EDGE ( 'NONE', *, *, #16992, .T. ) ;
#23780=VECTOR ( 'NONE', #35994, 999.9999999999998863 ) ;
#23812=VERTEX_POINT ( 'NONE', #35729 ) ;
#23813=VECTOR ( 'NONE', #1280, 999.9999999999998863 ) ;
#23820=CIRCLE ( 'NONE', #1241, 2.999999999999999556 ) ;
#23825=DIRECTION ( 'NONE',  ( -0.7871354856660162103, -0.4483307682966942709, -0.4235767337848251879 ) ) ;
#23839=CARTESIAN_POINT ( 'NONE',  ( 70.19189222814998175, -100.0979043305785581, -53.24182196210380624 ) ) ;
#23849=AXIS2_PLACEMENT_3D ( 'NONE', #42822, #29579, #11808 ) ;
#23851=CARTESIAN_POINT ( 'NONE',  ( 73.07463722459043254, -52.71812238298048214, -33.39556644922822670 ) ) ;
#23856=ADVANCED_FACE ( 'NONE', ( #19087 ), #35956, .T. ) ;
#23880=DIRECTION ( 'NONE',  ( -0.000000000000000000, -0.9284778069183721172, -0.3713878862591650232 ) ) ;
#23883=( LENGTH_UNIT ( ) NAMED_UNIT ( * ) SI_UNIT ( .MILLI., .METRE. ) );
#23895=CARTESIAN_POINT ( 'NONE',  ( 71.49305703095983233, -68.66289132450961574, -45.53212498594413660 ) ) ;
#23914=EDGE_LOOP ( 'NONE', ( #17417, #13491, #20997, #35372, #10145 ) ) ;
#23925=EDGE_CURVE ( 'NONE', #1444, #39549, #2154, .T. ) ;
#23942=CARTESIAN_POINT ( 'NONE',  ( 70.19189222814998175, -54.26662894631272849, -34.90947156805651019 ) ) ;
#23944=CARTESIAN_POINT ( 'NONE',  ( 70.19189222814998175, -67.83330054016514055, -40.33609291459782753 ) ) ;
#23956=CARTESIAN_POINT ( 'NONE',  ( 70.19189222814998175, -53.54563792646638376, -34.62107767336419073 ) ) ;
#23958=VERTEX_POINT ( 'NONE', #42819 ) ;
#23959=LINE ( 'NONE', #17116, #2291 ) ;
#23976=DIRECTION ( 'NONE',  ( -0.000000000000000000, -0.9284778069183721172, -0.3713878862591650232 ) ) ;
#23989=LINE ( 'NONE', #27179, #26943 ) ;
#23992=EDGE_CURVE ( 'NONE', #23245, #44431, #33419, .T. ) ;
#24017=CARTESIAN_POINT ( 'NONE',  ( 69.36136150295220659, -55.33724551716493067, -32.23290681585656614 ) ) ;
#24028=AXIS2_PLACEMENT_3D ( 'NONE', #37837, #16888, #26911 ) ;
#24031=EDGE_LOOP ( 'NONE', ( #38908, #19859, #29780, #44623, #30733, #42040 ) ) ;
#24049=VECTOR ( 'NONE', #43518, 1000.000000000000114 ) ;
#24053=CARTESIAN_POINT ( 'NONE',  ( 72.54180985774836188, -54.15757082072580175, -34.13667568191001322 ) ) ;
#24054=VERTEX_POINT ( 'NONE', #19317 ) ;
#24057=AXIS2_PLACEMENT_3D ( 'NONE', #17493, #31177, #6566 ) ;
#24060=DIRECTION ( 'NONE',  ( 1.387778780781445676E-17, -0.9284778069183720062, -0.3713878862591650232 ) ) ;
#24064=AXIS2_PLACEMENT_3D ( 'NONE', #22349, #29865, #5681 ) ;
#24071=DIRECTION ( 'NONE',  ( -0.000000000000000000, -0.9284778069183721172, -0.3713878862591650232 ) ) ;
#24097=DIRECTION ( 'NONE',  ( -0.000000000000000000, -0.9284778069183718952, -0.3713878862591649677 ) ) ;
#24101=ADVANCED_FACE ( 'NONE', ( #30252 ), #21106, .T. ) ;
#24131=CARTESIAN_POINT ( 'NONE',  ( 71.02242295334774269, -99.02728775972636299, -55.91838671430374319 ) ) ;
#24139=CARTESIAN_POINT ( 'NONE',  ( 71.02242295334774269, -49.68958793485906256, -36.18347876678663511 ) ) ;
#24147=EDGE_LOOP ( 'NONE', ( #35830, #39970, #20242, #28684, #5615, #30243 ) ) ;
#24153=AXIS2_PLACEMENT_3D ( 'NONE', #8464, #22367, #12115 ) ;
#24182=ORIENTED_EDGE ( 'NONE', *, *, #2301, .F. ) ;
#24194=ADVANCED_FACE ( 'NONE', ( #6310 ), #44440, .T. ) ;
#24195=CARTESIAN_POINT ( 'NONE',  ( 67.30914723170953096, -55.81513550964497483, -36.42337668688479368 ) ) ;
#24222=EDGE_CURVE ( 'NONE', #12877, #219, #43944, .T. ) ;
#24232=DIRECTION ( 'NONE',  ( -0.000000000000000000, -0.9284778069183721172, -0.3713878862591650232 ) ) ;
#24237=DIRECTION ( 'NONE',  ( 0.9609149988134843001, -0.1028163501681632064, 0.2570431154366505933 ) ) ;
#24255=CIRCLE ( 'NONE', #8220, 2.999999999999999556 ) ;
#24272=DIRECTION ( 'NONE',  ( -0.000000000000000000, -0.9284778069183721172, -0.3713878862591650232 ) ) ;
#24289=ADVANCED_FACE ( 'NONE', ( #17257 ), #17690, .T. ) ;
#24297=DIRECTION ( 'NONE',  ( -0.000000000000000000, -0.9284778069183721172, -0.3713878862591650232 ) ) ;
#24331=DIRECTION ( 'NONE',  ( -0.000000000000000000, -0.9284778069183721172, -0.3713878862591650232 ) ) ;
#24332=CARTESIAN_POINT ( 'NONE',  ( 70.19189222814998175, -70.61873396092025246, -41.45025657337532010 ) ) ;
#24374=CARTESIAN_POINT ( 'NONE',  ( 70.19189222814998175, -56.33107134722149567, -35.73524133214168330 ) ) ;
#24376=CARTESIAN_POINT ( 'NONE',  ( 70.19189222814998175, -51.48119552555760947, -33.79530790927901052 ) ) ;
#24421=ORIENTED_EDGE ( 'NONE', *, *, #13048, .T. ) ;
#24427=DIRECTION ( 'NONE',  ( 0.2768435750659113959, 0.3568721902840756854, -0.8921882507333144252 ) ) ;
#24465=CIRCLE ( 'NONE', #10634, 5.000000000000002665 ) ;
#24486=EDGE_CURVE ( 'NONE', #26292, #17071, #21862, .T. ) ;
#24491=ADVANCED_FACE ( 'NONE', ( #19653 ), #8951, .T. ) ;
#24492=ORIENTED_EDGE ( 'NONE', *, *, #27807, .F. ) ;
#24498=CIRCLE ( 'NONE', #25961, 2.999999999999999556 ) ;
#24502=CARTESIAN_POINT ( 'NONE',  ( 70.19189222814998175, -52.04917782255280656, -34.02249884819201498 ) ) ;
#24510=FACE_OUTER_BOUND ( 'NONE', #5956, .T. ) ;
#24542=EDGE_CURVE ( 'NONE', #37423, #36514, #13866, .T. ) ;
#24548=DIRECTION ( 'NONE',  ( -0.2407039305251457151, 0.3604685577742790525, -0.9011792478113758165 ) ) ;
#24549=DIRECTION ( 'NONE',  ( -0.000000000000000000, -0.9284778069183721172, -0.3713878862591650232 ) ) ;
#24574=DIRECTION ( 'NONE',  ( 0.9609149988134839671, -0.1028163501681660097, 0.2570431154366504822 ) ) ;
#24599=EDGE_CURVE ( 'NONE', #23245, #39765, #20787, .T. ) ;
#24606=ORIENTED_EDGE ( 'NONE', *, *, #41775, .F. ) ;
#24613=ORIENTED_EDGE ( 'NONE', *, *, #3931, .T. ) ;
#24649=ADVANCED_FACE ( 'NONE', ( #3667 ), #16811, .F. ) ;
#24656=ORIENTED_EDGE ( 'NONE', *, *, #4774, .F. ) ;
#24687=ORIENTED_EDGE ( 'NONE', *, *, #11706, .T. ) ;
#24709=LINE ( 'NONE', #28592, #39270 ) ;
#24710=CONICAL_SURFACE ( 'NONE', #43653, 2.445500000000004448, 0.9599310885968757034 ) ;
#24740=ORIENTED_EDGE ( 'NONE', *, *, #3275, .F. ) ;
#24749=CARTESIAN_POINT ( 'NONE',  ( 70.19189222814998175, -50.70706315265230302, -33.48565765860439569 ) ) ;
#24761=CARTESIAN_POINT ( 'NONE',  ( 70.19189222814998175, -100.0979043305785581, -53.24182196210380624 ) ) ;
#24766=EDGE_LOOP ( 'NONE', ( #14324, #17028, #22640, #26871, #25370 ) ) ;
#24789=EDGE_LOOP ( 'NONE', ( #4529, #31517, #2826, #27099, #15553 ) ) ;
#24803=ORIENTED_EDGE ( 'NONE', *, *, #25873, .F. ) ;
#24810=VECTOR ( 'NONE', #6685, 1000.000000000000227 ) ;
#24830=CARTESIAN_POINT ( 'NONE',  ( 70.19189222814998175, -57.98054017398621340, -36.39502311309316696 ) ) ;
#24836=DIRECTION ( 'NONE',  ( -0.000000000000000000, -0.9284778069183721172, -0.3713878862591650232 ) ) ;
#24846=CIRCLE ( 'NONE', #5892, 2.999999999999999556 ) ;
#24900=ORIENTED_EDGE ( 'NONE', *, *, #5394, .F. ) ;
#24969=ORIENTED_EDGE ( 'NONE', *, *, #21716, .F. ) ;
#25036=DIRECTION ( 'NONE',  ( -0.000000000000000000, -0.9284778069183721172, -0.3713878862591650232 ) ) ;
#25043=EDGE_CURVE ( 'NONE', #12184, #21045, #38534, .T. ) ;
#25052=DIRECTION ( 'NONE',  ( -0.9609149988134837450, 0.1028163501681639419, -0.2570431154366518145 ) ) ;
#25059=CARTESIAN_POINT ( 'NONE',  ( 71.02242295334774269, -53.19601237546052630, -37.58603632025644714 ) ) ;
#25060=CARTESIAN_POINT ( 'NONE',  ( 70.19189222814998175, -61.90193818873174791, -37.96356864969668266 ) ) ;
#25061=CARTESIAN_POINT ( 'NONE',  ( 68.07789357685331311, -68.58957386525776201, -38.44539312525988350 ) ) ;
#25063=ORIENTED_EDGE ( 'NONE', *, *, #21716, .T. ) ;
#25091=CARTESIAN_POINT ( 'NONE',  ( 73.07463722459043254, -51.99713136313413031, -33.10717255453590013 ) ) ;
#25094=ORIENTED_EDGE ( 'NONE', *, *, #38936, .T. ) ;
#25099=AXIS2_PLACEMENT_3D ( 'NONE', #24376, #13450, #41048 ) ;
#25131=VECTOR ( 'NONE', #860, 1000.000000000000227 ) ;
#25147=CARTESIAN_POINT ( 'NONE',  ( 69.36136150295220659, -51.77767972350450520, -30.80909290640445519 ) ) ;
#25152=VERTEX_POINT ( 'NONE', #32598 ) ;
#25158=EDGE_LOOP ( 'NONE', ( #13682, #30742, #17332, #11349 ) ) ;
#25187=CIRCLE ( 'NONE', #34628, 2.445500000000004448 ) ;
#25199=EDGE_CURVE ( 'NONE', #8760, #18545, #19685, .T. ) ;
#25207=DIRECTION ( 'NONE',  ( -0.2768435750659243300, -0.3568721902840674698, 0.8921882507333136481 ) ) ;
#25214=DIRECTION ( 'NONE',  ( 0.9609149988134837450, -0.1028163501681639419, 0.2570431154366518145 ) ) ;
#25218=AXIS2_PLACEMENT_3D ( 'NONE', #41276, #30539, #30992 ) ;
#25219=CARTESIAN_POINT ( 'NONE',  ( 67.30914723170953096, -50.45175545520677929, -34.27804336089664616 ) ) ;
#25222=EDGE_CURVE ( 'NONE', #19524, #23245, #43711, .T. ) ;
#25259=DIRECTION ( 'NONE',  ( -0.000000000000000000, -0.9284778069183721172, -0.3713878862591650232 ) ) ;
#25267=DIRECTION ( 'NONE',  ( 0.000000000000000000, 0.9284778069183720062, 0.3713878862591650232 ) ) ;
#25285=ADVANCED_FACE ( 'NONE', ( #36910 ), #31326, .T. ) ;
#25288=FACE_OUTER_BOUND ( 'NONE', #44165, .T. ) ;
#25289=CARTESIAN_POINT ( 'NONE',  ( 69.36136150295220659, -59.97963455175678860, -34.08984624715239420 ) ) ;
#25298=EDGE_CURVE ( 'NONE', #13764, #8341, #4381, .T. ) ;
#25308=DIRECTION ( 'NONE',  ( -0.7871354856660162103, -0.4483307682966942709, -0.4235767337848251879 ) ) ;
#25313=CIRCLE ( 'NONE', #10029, 2.445500000000004448 ) ;
#25327=CYLINDRICAL_SURFACE ( 'NONE', #14219, 3.000000000000001776 ) ;
#25350=DIRECTION ( 'NONE',  ( 0.9609149988134837450, -0.1028163501681639419, 0.2570431154366518145 ) ) ;
#25370=ORIENTED_EDGE ( 'NONE', *, *, #21755, .T. ) ;
#25380=CIRCLE ( 'NONE', #42139, 2.445500000000001339 ) ;
#25406=LINE ( 'NONE', #11046, #30055 ) ;
#25409=DIRECTION ( 'NONE',  ( 0.9609149988134843001, -0.1028163501681632064, 0.2570431154366505933 ) ) ;
#25429=EDGE_CURVE ( 'NONE', #18421, #18481, #2036, .T. ) ;
#25441=CARTESIAN_POINT ( 'NONE',  ( 70.19189222814998175, -57.05206236706784040, -36.02363522683400276 ) ) ;
#25442=CARTESIAN_POINT ( 'NONE',  ( 70.19189222814998175, -55.40259354030312267, -35.36385344588251911 ) ) ;
#25458=FACE_OUTER_BOUND ( 'NONE', #9282, .T. ) ;
#25475=CONICAL_SURFACE ( 'NONE', #29826, 2.445500000000004448, 0.9599310885968757034 ) ;
#25485=VERTEX_POINT ( 'NONE', #16419 ) ;
#25499=CONICAL_SURFACE ( 'NONE', #2180, 2.999999999999999556, 0.9599310885968830309 ) ;
#25500=CARTESIAN_POINT ( 'NONE',  ( 68.80767435282035649, -101.8822652819988974, -48.78088070843723756 ) ) ;
#25507=ORIENTED_EDGE ( 'NONE', *, *, #27880, .T. ) ;
#25511=CARTESIAN_POINT ( 'NONE',  ( 70.19189222814998175, -59.83749578782295941, -37.13779888561150244 ) ) ;
#25512=VECTOR ( 'NONE', #2911, 1000.000000000000114 ) ;
#25543=VECTOR ( 'NONE', #27040, 1000.000000000000114 ) ;
#25554=CARTESIAN_POINT ( 'NONE',  ( 67.30914723170953096, -59.52904673731846685, -37.90892823192145755 ) ) ;
#25570=EDGE_CURVE ( 'NONE', #24054, #9778, #4413, .T. ) ;
#25572=DIRECTION ( 'NONE',  ( -0.000000000000000000, -0.9284778069183720062, -0.3713878862591650232 ) ) ;
#25573=FACE_BOUND ( 'NONE', #12362, .T. ) ;
#25578=CARTESIAN_POINT ( 'NONE',  ( 73.01241679510815175, -68.13509210538408922, -39.58160742654554554 ) ) ;
#25583=CIRCLE ( 'NONE', #39309, 2.999999999999999556 ) ;
#25614=FACE_OUTER_BOUND ( 'NONE', #16598, .T. ) ;
#25617=EDGE_CURVE ( 'NONE', #25152, #16121, #31361, .T. ) ;
#25626=DIRECTION ( 'NONE',  ( -0.6937550123170076466, 0.2674776663120608799, -0.6686999932026935767 ) ) ;
#25688=LINE ( 'NONE', #16098, #4376 ) ;
#25707=DIRECTION ( 'NONE',  ( -0.2768435750659241079, -0.3568721902840695792, 0.8921882507333129819 ) ) ;
#25729=LINE ( 'NONE', #7714, #16174 ) ;
#25731=EDGE_LOOP ( 'NONE', ( #14284, #39614, #3659 ) ) ;
#25752=( LENGTH_UNIT ( ) NAMED_UNIT ( * ) SI_UNIT ( .MILLI., .METRE. ) );
#25758=EDGE_CURVE ( 'NONE', #35202, #42996, #36488, .T. ) ;
#25767=ORIENTED_EDGE ( 'NONE', *, *, #20893, .T. ) ;
#25774=CARTESIAN_POINT ( 'NONE',  ( 70.19189222814998175, -55.40259354030312267, -35.36385344588251911 ) ) ;
#25797=ORIENTED_EDGE ( 'NONE', *, *, #6990, .T. ) ;
#25805=VERTEX_POINT ( 'NONE', #34580 ) ;
#25806=CIRCLE ( 'NONE', #14189, 2.999999999999999556 ) ;
#25810=VERTEX_POINT ( 'NONE', #19172 ) ;
#25829=CARTESIAN_POINT ( 'NONE',  ( 70.19189222814998175, -60.40547808481815650, -37.36498982452450690 ) ) ;
#25840=DIRECTION ( 'NONE',  ( -0.000000000000000000, -0.9284778069183721172, -0.3713878862591650232 ) ) ;
#25841=DIRECTION ( 'NONE',  ( 0.9609149988134843001, -0.1028163501681632064, 0.2570431154366505933 ) ) ;
#25848=ORIENTED_EDGE ( 'NONE', *, *, #8269, .T. ) ;
#25855=CARTESIAN_POINT ( 'NONE',  ( 71.02242295334774269, -52.26753456854214619, -37.21464843399728295 ) ) ;
#25867=ORIENTED_EDGE ( 'NONE', *, *, #39430, .F. ) ;
#25873=EDGE_CURVE ( 'NONE', #35202, #2361, #38450, .T. ) ;
#25874=ADVANCED_FACE ( 'NONE', ( #35242 ), #31615, .F. ) ;
#25875=EDGE_CURVE ( 'NONE', #20614, #18078, #29550, .T. ) ;
#25876=AXIS2_PLACEMENT_3D ( 'NONE', #7809, #35828, #32853 ) ;
#25877=DIRECTION ( 'NONE',  ( 0.000000000000000000, 0.9284778069183720062, 0.3713878862591650232 ) ) ;
#25885=CARTESIAN_POINT ( 'NONE',  ( 73.07463722459043254, -54.78256478388924933, -34.22133621331339981 ) ) ;
#25892=CIRCLE ( 'NONE', #12826, 2.445500000000004448 ) ;
#25917=VERTEX_POINT ( 'NONE', #8353 ) ;
#25919=AXIS2_PLACEMENT_3D ( 'NONE', #135, #34770, #3549 ) ;
#25939=DIRECTION ( 'NONE',  ( 0.7871354856660167654, -0.6167752151498625546, -0.002461946824136807422 ) ) ;
#25940=EDGE_CURVE ( 'NONE', #1444, #15917, #22641, .T. ) ;
#25961=AXIS2_PLACEMENT_3D ( 'NONE', #3035, #58, #13972 ) ;
#25964=ORIENTED_EDGE ( 'NONE', *, *, #32365, .F. ) ;
#25981=AXIS2_PLACEMENT_3D ( 'NONE', #28242, #25267, #10690 ) ;
#26009=ORIENTED_EDGE ( 'NONE', *, *, #17855, .T. ) ;
#26037=VERTEX_POINT ( 'NONE', #26128 ) ;
#26044=ORIENTED_EDGE ( 'NONE', *, *, #14805, .T. ) ;
#26049=ORIENTED_EDGE ( 'NONE', *, *, #8582, .T. ) ;
#26050=CARTESIAN_POINT ( 'NONE',  ( 71.02242295334774269, -99.02728775972636299, -55.91838671430374319 ) ) ;
#26053=VECTOR ( 'NONE', #23825, 999.9999999999998863 ) ;
#26068=FACE_OUTER_BOUND ( 'NONE', #31802, .T. ) ;
#26072=DIRECTION ( 'NONE',  ( 0.2407039305251456596, -0.3604685577742790525, 0.9011792478113757054 ) ) ;
#26085=ORIENTED_EDGE ( 'NONE', *, *, #32840, .T. ) ;
#26089=CONICAL_SURFACE ( 'NONE', #42106, 2.999999999999999556, 0.9599310885968830309 ) ;
#26128=CARTESIAN_POINT ( 'NONE',  ( 67.30914723170953096, -51.17274647505311691, -34.56643725558897273 ) ) ;
#26137=EDGE_CURVE ( 'NONE', #23958, #37519, #19710, .T. ) ;
#26158=FACE_OUTER_BOUND ( 'NONE', #24031, .T. ) ;
#26163=EDGE_CURVE ( 'NONE', #4027, #12184, #18834, .T. ) ;
#26183=VECTOR ( 'NONE', #34968, 1000.000000000000000 ) ;
#26200=DIRECTION ( 'NONE',  ( -0.000000000000000000, -0.9284778069183718952, -0.3713878862591649677 ) ) ;
#26206=ORIENTED_EDGE ( 'NONE', *, *, #796, .T. ) ;
#26213=CONICAL_SURFACE ( 'NONE', #43697, 2.999999999999999556, 0.9599310885968830309 ) ;
#26228=EDGE_CURVE ( 'NONE', #31092, #9213, #40859, .T. ) ;
#26235=FACE_OUTER_BOUND ( 'NONE', #14770, .T. ) ;
#26249=CYLINDRICAL_SURFACE ( 'NONE', #10185, 3.000000000000001776 ) ;
#26252=CARTESIAN_POINT ( 'NONE',  ( 71.02242295334774269, -99.02728775972636299, -55.91838671430374319 ) ) ;
#26256=ORIENTED_EDGE ( 'NONE', *, *, #14510, .T. ) ;
#26262=VERTEX_POINT ( 'NONE', #35766 ) ;
#26263=VECTOR ( 'NONE', #22125, 1000.000000000000227 ) ;
#26269=ORIENTED_EDGE ( 'NONE', *, *, #25758, .T. ) ;
#26274=ORIENTED_EDGE ( 'NONE', *, *, #216, .F. ) ;
#26288=AXIS2_PLACEMENT_3D ( 'NONE', #44946, #31236, #36995 ) ;
#26289=FACE_OUTER_BOUND ( 'NONE', #25158, .T. ) ;
#26292=VERTEX_POINT ( 'NONE', #8193 ) ;
#26321=AXIS2_PLACEMENT_3D ( 'NONE', #15300, #8008, #36037 ) ;
#26380=ORIENTED_EDGE ( 'NONE', *, *, #1583, .F. ) ;
#26388=CARTESIAN_POINT ( 'NONE',  ( 69.36136150295220659, -57.40168791807370496, -33.05867657994173925 ) ) ;
#26390=EDGE_CURVE ( 'NONE', #42481, #4027, #35989, .T. ) ;
#26393=CARTESIAN_POINT ( 'NONE',  ( 69.36136150295220659, -101.1685209014307674, -50.56525720990386219 ) ) ;
#26408=AXIS2_PLACEMENT_3D ( 'NONE', #35646, #42285, #4420 ) ;
#26412=ORIENTED_EDGE ( 'NONE', *, *, #21755, .F. ) ;
#26416=ORIENTED_EDGE ( 'NONE', *, *, #2764, .F. ) ;
#26454=DIRECTION ( 'NONE',  ( 0.9609149988134843001, -0.1028163501681632064, 0.2570431154366505933 ) ) ;
#26491=CIRCLE ( 'NONE', #6830, 2.999999999999999556 ) ;
#26504=DIRECTION ( 'NONE',  ( -0.000000000000000000, -0.9284778069183718952, -0.3713878862591649677 ) ) ;
#26514=VERTEX_POINT ( 'NONE', #21860 ) ;
#26531=CARTESIAN_POINT ( 'NONE',  ( 67.84197459855160162, -58.29708508664516842, -37.25081299080650865 ) ) ;
#26604=DIRECTION ( 'NONE',  ( 0.9609149988134837450, -0.1028163501681639419, 0.2570431154366518145 ) ) ;
#26606=ORIENTED_EDGE ( 'NONE', *, *, #37137, .T. ) ;
#26611=EDGE_CURVE ( 'NONE', #6975, #16083, #39406, .T. ) ;
#26616=CARTESIAN_POINT ( 'NONE',  ( 67.37136766119182596, -67.53150897494617766, -41.09057840265009531 ) ) ;
#26623=ORIENTED_EDGE ( 'NONE', *, *, #3581, .F. ) ;
#26660=AXIS2_PLACEMENT_3D ( 'NONE', #8273, #1858, #31906 ) ;
#26673=DIRECTION ( 'NONE',  ( 0.7871354856660167654, -0.6167752151498625546, -0.002461946824136807422 ) ) ;
#26675=TOROIDAL_SURFACE ( 'NONE', #27406, 4.700000000000000178, 0.2999999999999999889 ) ;
#26696=VECTOR ( 'NONE', #33477, 1000.000000000000227 ) ;
#26704=CARTESIAN_POINT ( 'NONE',  ( 70.19189222814998175, -100.0979043305785581, -53.24182196210380624 ) ) ;
#26714=CIRCLE ( 'NONE', #16571, 2.999999999999999556 ) ;
#26716=ORIENTED_EDGE ( 'NONE', *, *, #216, .T. ) ;
#26759=ORIENTED_EDGE ( 'NONE', *, *, #22236, .F. ) ;
#26781=CONICAL_SURFACE ( 'NONE', #29668, 2.445500000000001339, 0.7853981633974680410 ) ;
#26803=EDGE_CURVE ( 'NONE', #21214, #3126, #237, .T. ) ;
#26809=DIRECTION ( 'NONE',  ( 0.7871354856660198740, 0.4483307682966886643, 0.4235767337848242442 ) ) ;
#26837=DIRECTION ( 'NONE',  ( 0.7871354856660167654, -0.6167752151498625546, -0.002461946824136807422 ) ) ;
#26864=DIRECTION ( 'NONE',  ( -0.000000000000000000, -0.9284778069183721172, -0.3713878862591650232 ) ) ;
#26871=ORIENTED_EDGE ( 'NONE', *, *, #9118, .T. ) ;
#26876=SURFACE_STYLE_FILL_AREA ( #20041 ) ;
#26889=CYLINDRICAL_SURFACE ( 'NONE', #34709, 3.000000000000001776 ) ;
#26892=LINE ( 'NONE', #26050, #40507 ) ;
#26898=CYLINDRICAL_SURFACE ( 'NONE', #34667, 3.000000000000001776 ) ;
#26907=ORIENTED_EDGE ( 'NONE', *, *, #11791, .F. ) ;
#26911=DIRECTION ( 'NONE',  ( 0.9609149988134843001, -0.1028163501681632064, 0.2570431154366505933 ) ) ;
#26934=CARTESIAN_POINT ( 'NONE',  ( 67.84197459855160162, -51.79774043821656448, -34.65109778699235221 ) ) ;
#26943=VECTOR ( 'NONE', #44966, 1000.000000000000114 ) ;
#26946=AXIS2_PLACEMENT_3D ( 'NONE', #4948, #1526, #14997 ) ;
#26949=LINE ( 'NONE', #33537, #18495 ) ;
#26977=CARTESIAN_POINT ( 'NONE',  ( 69.36136150295220659, -59.25864353191045808, -33.80145235246007474 ) ) ;
#26978=FACE_OUTER_BOUND ( 'NONE', #19473, .T. ) ;
#26986=AXIS2_PLACEMENT_3D ( 'NONE', #7094, #31040, #6878 ) ;
#26991=EDGE_CURVE ( 'NONE', #37423, #15070, #907, .T. ) ;
#26997=CYLINDRICAL_SURFACE ( 'NONE', #6305, 3.000000000000001776 ) ;
#26998=EDGE_CURVE ( 'NONE', #27773, #4363, #27676, .T. ) ;
#26999=EDGE_CURVE ( 'NONE', #39653, #32876, #25583, .T. ) ;
#27001=AXIS2_PLACEMENT_3D ( 'NONE', #42271, #14904, #32440 ) ;
#27004=DIRECTION ( 'NONE',  ( -0.000000000000000000, -0.9284778069183718952, -0.3713878862591649677 ) ) ;
#27008=DIRECTION ( 'NONE',  ( -0.000000000000000000, -0.9284778069183721172, -0.3713878862591650232 ) ) ;
#27018=EDGE_CURVE ( 'NONE', #35636, #25810, #23989, .T. ) ;
#27034=DIRECTION ( 'NONE',  ( -0.000000000000000000, -0.9284778069183718952, -0.3713878862591649677 ) ) ;
#27040=DIRECTION ( 'NONE',  ( 0.7202110682883375858, 0.2576522076061144029, -0.6441361323747234469 ) ) ;
#27064=EDGE_CURVE ( 'NONE', #25805, #3754, #41544, .T. ) ;
#27067=( NAMED_UNIT ( * ) PLANE_ANGLE_UNIT ( ) SI_UNIT ( $, .RADIAN. ) );
#27099=ORIENTED_EDGE ( 'NONE', *, *, #10044, .T. ) ;
#27101=DIRECTION ( 'NONE',  ( 0.7871354856660198740, 0.4483307682966886643, 0.4235767337848242442 ) ) ;
#27102=ORIENTED_EDGE ( 'NONE', *, *, #39833, .F. ) ;
#27112=ORIENTED_EDGE ( 'NONE', *, *, #33087, .T. ) ;
#27127=DIRECTION ( 'NONE',  ( -0.2768435750659241079, -0.3568721902840695792, 0.8921882507333129819 ) ) ;
#27145=ORIENTED_EDGE ( 'NONE', *, *, #1583, .T. ) ;
#27179=CARTESIAN_POINT ( 'NONE',  ( 70.89562859596755118, -66.92613143246303764, -42.60403544796190545 ) ) ;
#27181=DIRECTION ( 'NONE',  ( -0.000000000000000000, -0.9284778069183721172, -0.3713878862591650232 ) ) ;
#27210=DIRECTION ( 'NONE',  ( -0.000000000000000000, -0.9284778069183721172, -0.3713878862591650232 ) ) ;
#27232=AXIS2_PLACEMENT_3D ( 'NONE', #13527, #41357, #31063 ) ;
#27238=EDGE_LOOP ( 'NONE', ( #28929, #16347, #9369, #5191, #38303 ) ) ;
#27256=EDGE_LOOP ( 'NONE', ( #8155, #26380, #43443, #24421, #26044 ) ) ;
#27267=CARTESIAN_POINT ( 'NONE',  ( 70.19189222814998175, -58.18802696105826300, -36.47801710466001879 ) ) ;
#27294=CARTESIAN_POINT ( 'NONE',  ( 72.54180985774836188, -51.37213739997068984, -33.02251202313252065 ) ) ;
#27299=FACE_OUTER_BOUND ( 'NONE', #13092, .T. ) ;
#27304=CARTESIAN_POINT ( 'NONE',  ( 70.19189222814998175, -61.33395589173652951, -37.73637771078367109 ) ) ;
#27307=ORIENTED_EDGE ( 'NONE', *, *, #6990, .F. ) ;
#27310=DIRECTION ( 'NONE',  ( -0.000000000000000000, -0.9284778069183718952, -0.3713878862591649677 ) ) ;
#27329=EDGE_LOOP ( 'NONE', ( #35392, #43830, #13068, #42022, #37714 ) ) ;
#27332=EDGE_LOOP ( 'NONE', ( #12706, #20297, #16263, #20489, #16994, #5428 ) ) ;
#27349=ORIENTED_EDGE ( 'NONE', *, *, #13318, .F. ) ;
#27355=FACE_OUTER_BOUND ( 'NONE', #22093, .T. ) ;
#27364=VERTEX_POINT ( 'NONE', #43776 ) ;
#27368=DIRECTION ( 'NONE',  ( -0.9609149988134837450, 0.1028163501681639419, -0.2570431154366518145 ) ) ;
#27379=AXIS2_PLACEMENT_3D ( 'NONE', #23944, #38265, #38053 ) ;
#27406=AXIS2_PLACEMENT_3D ( 'NONE', #6510, #37963, #6740 ) ;
#27455=CARTESIAN_POINT ( 'NONE',  ( 70.19189222814998175, -100.0979043305785581, -53.24182196210380624 ) ) ;
#27471=FACE_OUTER_BOUND ( 'NONE', #23583, .T. ) ;
#27473=CARTESIAN_POINT ( 'NONE',  ( 70.19189222814998175, -70.34019061884472990, -41.33884020749756871 ) ) ;
#27475=AXIS2_PLACEMENT_3D ( 'NONE', #40991, #34119, #40298 ) ;
#27478=DIRECTION ( 'NONE',  ( -0.2768435750659253847, -0.3568721902840677473, 0.8921882507333133150 ) ) ;
#27508=EDGE_LOOP ( 'NONE', ( #16306, #9545, #37106, #347, #68 ) ) ;
#27512=CARTESIAN_POINT ( 'NONE',  ( 70.19189222814998175, -50.19222220871606766, -33.27972307567368659 ) ) ;
#27526=CARTESIAN_POINT ( 'NONE',  ( 73.07463722459043254, -61.28190943231786036, -36.82105141712754914 ) ) ;
#27528=AXIS2_PLACEMENT_3D ( 'NONE', #23895, #3352, #6551 ) ;
#27529=CARTESIAN_POINT ( 'NONE',  ( 70.19189222814998175, -56.33107134722149567, -35.73524133214168330 ) ) ;
#27531=EDGE_CURVE ( 'NONE', #14756, #43396, #42981, .T. ) ;
#27553=ORIENTED_EDGE ( 'NONE', *, *, #6097, .T. ) ;
#27555=ORIENTED_EDGE ( 'NONE', *, *, #27531, .F. ) ;
#27564=AXIS2_PLACEMENT_3D ( 'NONE', #43754, #39651, #1780 ) ;
#27592=ORIENTED_EDGE ( 'NONE', *, *, #4467, .F. ) ;
#27600=DIRECTION ( 'NONE',  ( -0.000000000000000000, -0.9284778069183720062, -0.3713878862591650232 ) ) ;
#27616=EDGE_LOOP ( 'NONE', ( #41758, #25063, #18123, #33800, #20338 ) ) ;
#27626=VERTEX_POINT ( 'NONE', #6825 ) ;
#27634=DIRECTION ( 'NONE',  ( -0.000000000000000000, -0.9284778069183718952, -0.3713878862591649677 ) ) ;
#27636=CARTESIAN_POINT ( 'NONE',  ( 73.07463722459043254, -53.85408697697087632, -33.84994832705423562 ) ) ;
#27655=CARTESIAN_POINT ( 'NONE',  ( 70.19189222814998175, -55.40259354030312267, -35.36385344588251911 ) ) ;
#27661=CARTESIAN_POINT ( 'NONE',  ( 70.19189222814998175, -100.0979043305785581, -53.24182196210380624 ) ) ;
#27676=CIRCLE ( 'NONE', #43777, 2.445500000000004448 ) ;
#27681=CARTESIAN_POINT ( 'NONE',  ( 73.07463722459043254, -52.92560917005250332, -33.47856044079506432 ) ) ;
#27691=AXIS2_PLACEMENT_3D ( 'NONE', #23504, #13467, #33966 ) ;
#27697=DIRECTION ( 'NONE',  ( 0.000000000000000000, 0.9284778069183721172, 0.3713878862591650232 ) ) ;
#27722=DIRECTION ( 'NONE',  ( -0.2768435750659241079, -0.3568721902840686355, 0.8921882507333134260 ) ) ;
#27734=AXIS2_PLACEMENT_3D ( 'NONE', #7625, #28614, #3751 ) ;
#27752=FACE_OUTER_BOUND ( 'NONE', #36579, .T. ) ;
#27755=ORIENTED_EDGE ( 'NONE', *, *, #20936, .F. ) ;
#27773=VERTEX_POINT ( 'NONE', #4583 ) ;
#27784=ORIENTED_EDGE ( 'NONE', *, *, #39061, .T. ) ;
#27799=FACE_OUTER_BOUND ( 'NONE', #34190, .T. ) ;
#27807=EDGE_CURVE ( 'NONE', #42996, #23812, #11447, .T. ) ;
#27817=CARTESIAN_POINT ( 'NONE',  ( 70.19189222814998175, -67.83330054016514055, -40.33609291459782753 ) ) ;
#27829=CARTESIAN_POINT ( 'NONE',  ( 72.54180985774836188, -56.94300424148091366, -35.25083934068751290 ) ) ;
#27834=ADVANCED_FACE ( 'NONE', ( #36039 ), #7303, .T. ) ;
#27844=EDGE_CURVE ( 'NONE', #10287, #44451, #34223, .T. ) ;
#27854=CARTESIAN_POINT ( 'NONE',  ( 69.36136150295220659, -101.1685209014307674, -50.56525720990386219 ) ) ;
#27856=CARTESIAN_POINT ( 'NONE',  ( 70.19189222814998175, -64.81574766768041229, -39.12908228425553858 ) ) ;
#27858=LINE ( 'NONE', #3228, #40459 ) ;
#27866=DIRECTION ( 'NONE',  ( -0.000000000000000000, -0.9284778069183721172, -0.3713878862591650232 ) ) ;
#27880=EDGE_CURVE ( 'NONE', #36176, #36279, #8028, .T. ) ;
#27883=ORIENTED_EDGE ( 'NONE', *, *, #4774, .T. ) ;
#27886=CIRCLE ( 'NONE', #10437, 2.999999999999999556 ) ;
#27895=DIRECTION ( 'NONE',  ( -0.7871354856660202071, 0.6167752151498580027, 0.002461946824133919541 ) ) ;
#27896=AXIS2_PLACEMENT_3D ( 'NONE', #11974, #25877, #4889 ) ;
#27899=ORIENTED_EDGE ( 'NONE', *, *, #39791, .T. ) ;
#27912=DIRECTION ( 'NONE',  ( -0.000000000000000000, -0.9284778069183718952, -0.3713878862591649677 ) ) ;
#27915=CIRCLE ( 'NONE', #36637, 2.999999999999999556 ) ;
#27926=CARTESIAN_POINT ( 'NONE',  ( 72.54180985774836188, -56.01452643456254776, -34.87945145442834871 ) ) ;
#27961=DIRECTION ( 'NONE',  ( -0.2768435750659266059, -0.3568721902840680249, 0.8921882507333128709 ) ) ;
#27971=CARTESIAN_POINT ( 'NONE',  ( 69.36136150295220659, -61.11559914574721120, -34.54422812497841022 ) ) ;
#27976=DIRECTION ( 'NONE',  ( -0.2768435750659263839, -0.3568721902840679139, 0.8921882507333128709 ) ) ;
#28031=CONICAL_SURFACE ( 'NONE', #34551, 2.445500000000004448, 0.9599310885968757034 ) ;
#28038=DIRECTION ( 'NONE',  ( 0.9609149988134837450, -0.1028163501681639419, 0.2570431154366518145 ) ) ;
#28040=ORIENTED_EDGE ( 'NONE', *, *, #32038, .T. ) ;
#28055=CARTESIAN_POINT ( 'NONE',  ( 70.19189222814998175, -55.40259354030312267, -35.36385344588251911 ) ) ;
#28058=EDGE_LOOP ( 'NONE', ( #20467, #8556, #11376, #33414, #25964 ) ) ;
#28060=CARTESIAN_POINT ( 'NONE',  ( 70.19189222814998175, -100.0979043305785581, -53.24182196210380624 ) ) ;
#28070=VERTEX_POINT ( 'NONE', #34583 ) ;
#28095=EDGE_CURVE ( 'NONE', #34215, #1783, #21858, .T. ) ;
#28101=EDGE_CURVE ( 'NONE', #10336, #22908, #23682, .T. ) ;
#28132=ORIENTED_EDGE ( 'NONE', *, *, #9520, .F. ) ;
#28146=AXIS2_PLACEMENT_3D ( 'NONE', #11049, #18787, #35418 ) ;
#28167=DIRECTION ( 'NONE',  ( -0.000000000000000000, -0.9284778069183718952, -0.3713878862591649677 ) ) ;
#28168=EDGE_CURVE ( 'NONE', #44499, #14756, #8743, .T. ) ;
#28171=EDGE_LOOP ( 'NONE', ( #19204, #16512, #39297, #31299, #20010 ) ) ;
#28174=CARTESIAN_POINT ( 'NONE',  ( 71.02242295334774269, -57.11741039020605371, -39.15458185685995574 ) ) ;
#28197=CARTESIAN_POINT ( 'NONE',  ( 67.37136766119182596, -67.53150897494617766, -41.09057840265009531 ) ) ;
#28209=CARTESIAN_POINT ( 'NONE',  ( 70.19189222814998175, -59.47700027789979060, -36.99360193826534271 ) ) ;
#28214=DIRECTION ( 'NONE',  ( 0.2768435750659264949, 0.3568721902840676363, -0.8921882507333129819 ) ) ;
#28216=CIRCLE ( 'NONE', #1962, 2.999999999999999556 ) ;
#28235=EDGE_LOOP ( 'NONE', ( #34754, #18973 ) ) ;
#28242=CARTESIAN_POINT ( 'NONE',  ( 70.19189222814998175, -51.68868231262963775, -33.87830190084585524 ) ) ;
#28260=DIRECTION ( 'NONE',  ( 0.9609149988134837450, -0.1028163501681639419, 0.2570431154366518145 ) ) ;
#28286=ORIENTED_EDGE ( 'NONE', *, *, #22760, .F. ) ;
#28287=DIRECTION ( 'NONE',  ( -0.7871354856660162103, -0.4483307682966942709, -0.4235767337848251879 ) ) ;
#28303=DIRECTION ( 'NONE',  ( -0.000000000000000000, -0.9284778069183721172, -0.3713878862591650232 ) ) ;
#28313=EDGE_LOOP ( 'NONE', ( #45103, #37526, #1306, #44290, #11685, #545 ) ) ;
#28333=LINE ( 'NONE', #34915, #9620 ) ;
#28335=DIRECTION ( 'NONE',  ( -0.000000000000000000, -0.9284778069183718952, -0.3713878862591649677 ) ) ;
#28345=DIRECTION ( 'NONE',  ( -0.000000000000000000, -0.9284778069183720062, -0.3713878862591650232 ) ) ;
#28358=DIRECTION ( 'NONE',  ( 0.7871354856660198740, 0.4483307682966886643, 0.4235767337848242442 ) ) ;
#28361=CIRCLE ( 'NONE', #29111, 2.999999999999999556 ) ;
#28383=CARTESIAN_POINT ( 'NONE',  ( 70.19189222814998175, -60.04498257489500190, -37.22079287717834717 ) ) ;
#28393=ORIENTED_EDGE ( 'NONE', *, *, #41493, .F. ) ;
#28400=EDGE_CURVE ( 'NONE', #25805, #19894, #25688, .T. ) ;
#28405=DIRECTION ( 'NONE',  ( -0.000000000000000000, -0.9284778069183718952, -0.3713878862591649677 ) ) ;
#28414=CARTESIAN_POINT ( 'NONE',  ( 70.19189222814998175, -54.83461124330791847, -35.13666250696951465 ) ) ;
#28432=VECTOR ( 'NONE', #28358, 1000.000000000000227 ) ;
#28449=AXIS2_PLACEMENT_3D ( 'NONE', #22852, #36743, #5511 ) ;
#28476=AXIS2_PLACEMENT_3D ( 'NONE', #19375, #33719, #33483 ) ;
#28480=CARTESIAN_POINT ( 'NONE',  ( 69.36136150295220659, -62.76506797251190051, -35.20400990592987966 ) ) ;
#28487=CARTESIAN_POINT ( 'NONE',  ( 70.19189222814998175, -51.48119552555760947, -33.79530790927901052 ) ) ;
#28505=CYLINDRICAL_SURFACE ( 'NONE', #20595, 3.000000000000001776 ) ;
#28512=AXIS2_PLACEMENT_3D ( 'NONE', #29486, #43177, #25841 ) ;
#28528=CARTESIAN_POINT ( 'NONE',  ( 70.19189222814998175, -56.12358456014947450, -35.65224734057483857 ) ) ;
#28537=CARTESIAN_POINT ( 'NONE',  ( 71.02242295334774269, -56.18893258328766649, -38.78319397060078444 ) ) ;
#28580=ORIENTED_EDGE ( 'NONE', *, *, #3550, .T. ) ;
#28592=CARTESIAN_POINT ( 'NONE',  ( 73.07463722459043254, -58.49647601156275556, -35.70688775835006368 ) ) ;
#28600=PRODUCT_DEFINITION_FORMATION_WITH_SPECIFIED_SOURCE ( 'ANY', '', #28885, .NOT_KNOWN. ) ;
#28614=DIRECTION ( 'NONE',  ( -0.000000000000000000, -0.9284778069183721172, -0.3713878862591650232 ) ) ;
#28632=CIRCLE ( 'NONE', #35869, 2.999999999999999556 ) ;
#28636=CARTESIAN_POINT ( 'NONE',  ( 70.19189222814998175, -58.18802696105826300, -36.47801710466001879 ) ) ;
#28637=DIRECTION ( 'NONE',  ( 0.9609149988134837450, -0.1028163501681639419, 0.2570431154366518145 ) ) ;
#28642=DIRECTION ( 'NONE',  ( -0.000000000000000000, -0.9284778069183721172, -0.3713878862591650232 ) ) ;
#28684=ORIENTED_EDGE ( 'NONE', *, *, #11741, .T. ) ;
#28690=DIRECTION ( 'NONE',  ( 0.9609149988134837450, -0.1028163501681639419, 0.2570431154366518145 ) ) ;
#28698=EDGE_CURVE ( 'NONE', #1665, #44682, #19969, .T. ) ;
#28704=DIRECTION ( 'NONE',  ( -0.000000000000000000, -0.9284778069183718952, -0.3713878862591649677 ) ) ;
#28711=CARTESIAN_POINT ( 'NONE',  ( 70.19189222814998175, -54.47411573338475677, -34.99246555962335492 ) ) ;
#28714=CARTESIAN_POINT ( 'NONE',  ( 67.84197459855160162, -62.01099631431865333, -38.73636453584316541 ) ) ;
#28776=CONICAL_SURFACE ( 'NONE', #2555, 2.999999999999999556, 0.9599310885968830309 ) ;
#28782=DIRECTION ( 'NONE',  ( -0.000000000000000000, -0.9284778069183721172, -0.3713878862591650232 ) ) ;
#28797=ORIENTED_EDGE ( 'NONE', *, *, #34504, .F. ) ;
#28798=ORIENTED_EDGE ( 'NONE', *, *, #25617, .F. ) ;
#28819=EDGE_LOOP ( 'NONE', ( #42620, #7692, #37798, #28040, #26907, #44676 ) ) ;
#28827=CARTESIAN_POINT ( 'NONE',  ( 69.36136150295220659, -56.47321011115533196, -32.68728869368257506 ) ) ;
#28852=DIRECTION ( 'NONE',  ( -0.2768435750659113959, -0.3568721902840756854, 0.8921882507333144252 ) ) ;
#28885=PRODUCT ( 'Clamp Bolt', 'Clamp Bolt', '', ( #39149 ) ) ;
#28896=AXIS2_PLACEMENT_3D ( 'NONE', #2129, #19932, #33818 ) ;
#28919=DIRECTION ( 'NONE',  ( -0.000000000000000000, -0.9284778069183721172, -0.3713878862591650232 ) ) ;
#28922=AXIS2_PLACEMENT_3D ( 'NONE', #43487, #39837, #26604 ) ;
#28929=ORIENTED_EDGE ( 'NONE', *, *, #38276, .F. ) ;
#28943=ADVANCED_FACE ( 'NONE', ( #22709 ), #10253, .T. ) ;
#28949=CARTESIAN_POINT ( 'NONE',  ( 70.19189222814998175, -100.0979043305785581, -53.24182196210380624 ) ) ;
#28950=CARTESIAN_POINT ( 'NONE',  ( 67.84197459855160162, -52.72621824513493038, -35.02248567325151640 ) ) ;
#28989=ORIENTED_EDGE ( 'NONE', *, *, #34052, .F. ) ;
#28991=CARTESIAN_POINT ( 'NONE',  ( 70.19189222814998175, -56.69156685714467159, -35.87943827948784303 ) ) ;
#28992=CARTESIAN_POINT ( 'NONE',  ( 72.54180985774836188, -53.22909301380743585, -33.76528779565084903 ) ) ;
#29000=DIRECTION ( 'NONE',  ( -0.000000000000000000, -0.9284778069183721172, -0.3713878862591650232 ) ) ;
#29007=ORIENTED_EDGE ( 'NONE', *, *, #11389, .F. ) ;
#29009=DIRECTION ( 'NONE',  ( -0.7871354856660202071, 0.6167752151498580027, 0.002461946824133919541 ) ) ;
#29032=VERTEX_POINT ( 'NONE', #13588 ) ;
#29097=DIRECTION ( 'NONE',  ( 0.9609149988134837450, -0.1028163501681639419, 0.2570431154366518145 ) ) ;
#29111=AXIS2_PLACEMENT_3D ( 'NONE', #12243, #5602, #22713 ) ;
#29125=VERTEX_POINT ( 'NONE', #16563 ) ;
#29135=CIRCLE ( 'NONE', #27691, 2.445500000000004448 ) ;
#29144=VERTEX_POINT ( 'NONE', #17017 ) ;
#29167=EDGE_CURVE ( 'NONE', #34887, #26514, #30655, .T. ) ;
#29177=DIRECTION ( 'NONE',  ( 1.387778780781445676E-17, -0.9284778069183720062, -0.3713878862591650232 ) ) ;
#29197=VERTEX_POINT ( 'NONE', #45051 ) ;
#29216=VERTEX_POINT ( 'NONE', #4202 ) ;
#29229=EDGE_CURVE ( 'NONE', #9699, #42672, #10962, .T. ) ;
#29239=ORIENTED_EDGE ( 'NONE', *, *, #45138, .T. ) ;
#29247=LINE ( 'NONE', #15338, #20841 ) ;
#29249=CONICAL_SURFACE ( 'NONE', #5938, 2.445500000000004448, 0.9599310885968757034 ) ;
#29254=CARTESIAN_POINT ( 'NONE',  ( 70.19189222814998175, -64.81574766768041229, -39.12908228425553858 ) ) ;
#29271=CARTESIAN_POINT ( 'NONE',  ( 67.30914723170953096, -52.30871106904351819, -35.02081913341498165 ) ) ;
#29288=EDGE_CURVE ( 'NONE', #34097, #15244, #16805, .T. ) ;
#29298=CARTESIAN_POINT ( 'NONE',  ( 71.02242295334774269, -53.40349916253254747, -37.66903031182329897 ) ) ;
#29302=CARTESIAN_POINT ( 'NONE',  ( 70.19189222814998175, -53.90613343638955968, -34.76527462071035046 ) ) ;
#29312=EDGE_LOOP ( 'NONE', ( #8682, #2537, #3856, #8699, #6920, #27349 ) ) ;
#29334=LINE ( 'NONE', #19301, #30119 ) ;
#29352=EDGE_LOOP ( 'NONE', ( #12314, #36361, #8282, #21775, #35303, #1732 ) ) ;
#29356=LINE ( 'NONE', #43271, #36787 ) ;
#29363=AXIS2_PLACEMENT_3D ( 'NONE', #42803, #15202, #42353 ) ;
#29405=AXIS2_PLACEMENT_3D ( 'NONE', #35170, #41829, #7597 ) ;
#29414=DIRECTION ( 'NONE',  ( 0.9609149988134843001, -0.1028163501681632064, 0.2570431154366505933 ) ) ;
#29432=DIRECTION ( 'NONE',  ( -0.000000000000000000, -0.9284778069183721172, -0.3713878862591650232 ) ) ;
#29437=ORIENTED_EDGE ( 'NONE', *, *, #42324, .T. ) ;
#29443=LINE ( 'NONE', #26252, #10469 ) ;
#29451=ORIENTED_EDGE ( 'NONE', *, *, #30678, .T. ) ;
#29454=CIRCLE ( 'NONE', #37467, 2.999999999999999556 ) ;
#29455=ADVANCED_FACE ( 'NONE', ( #10615 ), #32240, .T. ) ;
#29478=AXIS2_PLACEMENT_3D ( 'NONE', #44456, #20061, #44236 ) ;
#29486=CARTESIAN_POINT ( 'NONE',  ( 70.19189222814998175, -55.76308905022629858, -35.50805039322867884 ) ) ;
#29489=CARTESIAN_POINT ( 'NONE',  ( 67.37136766119182596, -67.53150897494617766, -41.09057840265009531 ) ) ;
#29509=ORIENTED_EDGE ( 'NONE', *, *, #44007, .T. ) ;
#29513=CIRCLE ( 'NONE', #36073, 0.2499999999999990841 ) ;
#29527=ADVANCED_FACE ( 'NONE', ( #33345 ), #43773, .T. ) ;
#29550=LINE ( 'NONE', #39592, #3701 ) ;
#29560=CIRCLE ( 'NONE', #40466, 2.445500000000004448 ) ;
#29579=DIRECTION ( 'NONE',  ( -0.000000000000000000, -0.9284778069183721172, -0.3713878862591650232 ) ) ;
#29590=ORIENTED_EDGE ( 'NONE', *, *, #44006, .F. ) ;
#29604=ORIENTED_EDGE ( 'NONE', *, *, #29167, .T. ) ;
#29611=VERTEX_POINT ( 'NONE', #25855 ) ;
#29668=AXIS2_PLACEMENT_3D ( 'NONE', #11491, #4410, #43616 ) ;
#29685=ORIENTED_EDGE ( 'NONE', *, *, #8870, .F. ) ;
#29688=CARTESIAN_POINT ( 'NONE',  ( 70.19189222814998175, -57.25954915413987578, -36.10662921840084749 ) ) ;
#29721=CARTESIAN_POINT ( 'NONE',  ( 70.19189222814998175, -58.18802696105826300, -36.47801710466001879 ) ) ;
#29740=DIRECTION ( 'NONE',  ( -0.000000000000000000, -0.9284778069183720062, -0.3713878862591650232 ) ) ;
#29748=VERTEX_POINT ( 'NONE', #22656 ) ;
#29749=LINE ( 'NONE', #25885, #14203 ) ;
#29780=ORIENTED_EDGE ( 'NONE', *, *, #24222, .T. ) ;
#29781=DIRECTION ( 'NONE',  ( -0.000000000000000000, -0.9284778069183720062, -0.3713878862591650232 ) ) ;
#29794=AXIS2_PLACEMENT_3D ( 'NONE', #838, #35482, #24574 ) ;
#29798=ORIENTED_EDGE ( 'NONE', *, *, #28095, .T. ) ;
#29826=AXIS2_PLACEMENT_3D ( 'NONE', #6204, #30601, #41338 ) ;
#29835=FACE_OUTER_BOUND ( 'NONE', #11565, .T. ) ;
#29848=ADVANCED_FACE ( 'NONE', ( #38079 ), #30693, .T. ) ;
#29850=DIRECTION ( 'NONE',  ( -0.2768435750659239414, -0.3568721902840664151, 0.8921882507333142032 ) ) ;
#29865=DIRECTION ( 'NONE',  ( -0.000000000000000000, -0.9284778069183721172, -0.3713878862591650232 ) ) ;
#29875=ORIENTED_EDGE ( 'NONE', *, *, #40181, .T. ) ;
#29888=EDGE_CURVE ( 'NONE', #25152, #29197, #9209, .T. ) ;
#29897=DIRECTION ( 'NONE',  ( -0.000000000000000000, -0.9284778069183718952, -0.3713878862591649677 ) ) ;
#29924=EDGE_CURVE ( 'NONE', #9778, #1762, #2119, .T. ) ;
#29954=DIRECTION ( 'NONE',  ( -0.000000000000000000, -0.9284778069183718952, -0.3713878862591649677 ) ) ;
#29958=ORIENTED_EDGE ( 'NONE', *, *, #37559, .T. ) ;
#29966=CIRCLE ( 'NONE', #16868, 2.999999999999999556 ) ;
#29983=AXIS2_PLACEMENT_3D ( 'NONE', #42192, #23976, #3209 ) ;
#30017=EDGE_CURVE ( 'NONE', #4387, #12877, #2254, .T. ) ;
#30032=FACE_OUTER_BOUND ( 'NONE', #24789, .T. ) ;
#30055=VECTOR ( 'NONE', #41845, 1000.000000000000227 ) ;
#30065=MECHANICAL_DESIGN_GEOMETRIC_PRESENTATION_REPRESENTATION('',(#35187),#33689);
#30068=VERTEX_POINT ( 'NONE', #8420 ) ;
#30069=AXIS2_PLACEMENT_3D ( 'NONE', #31143, #20894, #34335 ) ;
#30089=CARTESIAN_POINT ( 'NONE',  ( 71.02242295334774269, -63.74513109682822432, -41.80564703645547553 ) ) ;
#30094=DIRECTION ( 'NONE',  ( -0.000000000000000000, -0.9284778069183721172, -0.3713878862591650232 ) ) ;
#30119=VECTOR ( 'NONE', #43692, 1000.000000000000227 ) ;
#30134=CIRCLE ( 'NONE', #23599, 2.999999999999999556 ) ;
#30164=EDGE_CURVE ( 'NONE', #32198, #29032, #38222, .T. ) ;
#30174=CARTESIAN_POINT ( 'NONE',  ( 70.19189222814998175, -58.18802696105826300, -36.47801710466001879 ) ) ;
#30198=CARTESIAN_POINT ( 'NONE',  ( 68.80767435282035649, -66.83222807083036798, -34.76098800215376627 ) ) ;
#30243=ORIENTED_EDGE ( 'NONE', *, *, #29167, .F. ) ;
#30252=FACE_OUTER_BOUND ( 'NONE', #34368, .T. ) ;
#30256=CARTESIAN_POINT ( 'NONE',  ( 70.19189222814998175, -60.04498257489500190, -37.22079287717834717 ) ) ;
#30265=ORIENTED_EDGE ( 'NONE', *, *, #26611, .F. ) ;
#30292=PRESENTATION_STYLE_ASSIGNMENT (( #41255 ) ) ;
#30303=VECTOR ( 'NONE', #12766, 1000.000000000000227 ) ;
#30314=CARTESIAN_POINT ( 'NONE',  ( 72.54180985774836188, -58.79995985531765967, -35.99361511320584128 ) ) ;
#30328=AXIS2_PLACEMENT_3D ( 'NONE', #24761, #367, #7884 ) ;
#30354=ADVANCED_FACE ( 'NONE', ( #20470 ), #7002, .T. ) ;
#30363=ADVANCED_FACE ( 'NONE', ( #37556 ), #29249, .T. ) ;
#30421=VECTOR ( 'NONE', #41382, 1000.000000000000227 ) ;
#30426=ORIENTED_EDGE ( 'NONE', *, *, #23727, .T. ) ;
#30429=CARTESIAN_POINT ( 'NONE',  ( 72.54180985774836188, -61.58539327607277869, -37.10777877198333385 ) ) ;
#30439=CARTESIAN_POINT ( 'NONE',  ( 68.07789357685331311, -68.58957386525776201, -38.44539312525988350 ) ) ;
#30461=VERTEX_POINT ( 'NONE', #12167 ) ;
#30471=EDGE_CURVE ( 'NONE', #36514, #37423, #123, .T. ) ;
#30486=FACE_OUTER_BOUND ( 'NONE', #27332, .T. ) ;
#30539=DIRECTION ( 'NONE',  ( 0.000000000000000000, 0.9284778069183720062, 0.3713878862591650232 ) ) ;
#30552=CARTESIAN_POINT ( 'NONE',  ( 67.30914723170953096, -55.09414448979863010, -36.13498279219247422 ) ) ;
#30560=ADVANCED_FACE ( 'NONE', ( #5751 ), #44086, .T. ) ;
#30586=ORIENTED_EDGE ( 'NONE', *, *, #37559, .F. ) ;
#30597=FACE_OUTER_BOUND ( 'NONE', #27616, .T. ) ;
#30601=DIRECTION ( 'NONE',  ( -0.000000000000000000, -0.9284778069183720062, -0.3713878862591650232 ) ) ;
#30636=ORIENTED_EDGE ( 'NONE', *, *, #35560, .T. ) ;
#30653=EDGE_CURVE ( 'NONE', #25917, #13764, #16902, .T. ) ;
#30655=CIRCLE ( 'NONE', #5115, 2.999999999999999556 ) ;
#30678=EDGE_CURVE ( 'NONE', #20119, #41097, #21955, .T. ) ;
#30693=CONICAL_SURFACE ( 'NONE', #8812, 2.999999999999999556, 0.9599310885968830309 ) ;
#30704=CARTESIAN_POINT ( 'NONE',  ( 69.36136150295220659, -101.1685209014307674, -50.56525720990386219 ) ) ;
#30733=ORIENTED_EDGE ( 'NONE', *, *, #14510, .F. ) ;
#30734=DIRECTION ( 'NONE',  ( -0.000000000000000000, -0.9284778069183721172, -0.3713878862591650232 ) ) ;
#30742=ORIENTED_EDGE ( 'NONE', *, *, #40253, .T. ) ;
#30746=( NAMED_UNIT ( * ) SI_UNIT ( $, .STERADIAN. ) SOLID_ANGLE_UNIT ( ) );
#30799=CARTESIAN_POINT ( 'NONE',  ( 70.19189222814998175, -67.83330054016514055, -40.33609291459782753 ) ) ;
#30810=DIRECTION ( 'NONE',  ( -0.7871354856660202071, 0.6167752151498580027, 0.002461946824133919541 ) ) ;
#30847=LINE ( 'NONE', #16500, #24810 ) ;
#30863=LINE ( 'NONE', #17408, #22978 ) ;
#30870=EDGE_CURVE ( 'NONE', #4363, #34274, #14180, .T. ) ;
#30876=DIRECTION ( 'NONE',  ( 0.9609149988134843001, -0.1028163501681632064, 0.2570431154366505933 ) ) ;
#30877=CARTESIAN_POINT ( 'NONE',  ( 67.30914723170953096, -52.30871106904351819, -35.02081913341498165 ) ) ;
#30885=CARTESIAN_POINT ( 'NONE',  ( 70.19189222814998175, -56.33107134722149567, -35.73524133214168330 ) ) ;
#30925=ORIENTED_EDGE ( 'NONE', *, *, #18739, .T. ) ;
#30928=EDGE_CURVE ( 'NONE', #40557, #39765, #29966, .T. ) ;
#30929=CIRCLE ( 'NONE', #34523, 2.999999999999999556 ) ;
#30946=CARTESIAN_POINT ( 'NONE',  ( 69.36136150295220659, -101.1685209014307674, -50.56525720990386219 ) ) ;
#30952=CONICAL_SURFACE ( 'NONE', #36753, 2.999999999999999556, 0.9599310885968830309 ) ;
#30966=EDGE_LOOP ( 'NONE', ( #4852, #41015, #15297, #5199, #4682 ) ) ;
#30988=EDGE_CURVE ( 'NONE', #32530, #33236, #12494, .T. ) ;
#30992=DIRECTION ( 'NONE',  ( -0.9609149988134837450, 0.1028163501681639419, -0.2570431154366518145 ) ) ;
#31040=DIRECTION ( 'NONE',  ( -0.000000000000000000, -0.9284778069183721172, -0.3713878862591650232 ) ) ;
#31050=CARTESIAN_POINT ( 'NONE',  ( 70.19189222814998175, -62.26243369865490251, -38.10776559704283528 ) ) ;
#31054=ADVANCED_FACE ( 'NONE', ( #15080 ), #825, .T. ) ;
#31063=DIRECTION ( 'NONE',  ( 0.9609149988134837450, -0.1028163501681639419, 0.2570431154366518145 ) ) ;
#31092=VERTEX_POINT ( 'NONE', #28992 ) ;
#31101=ORIENTED_EDGE ( 'NONE', *, *, #8582, .F. ) ;
#31102=CARTESIAN_POINT ( 'NONE',  ( 71.95541746945981743, -68.51322876793039995, -38.63625753187658063 ) ) ;
#31119=CARTESIAN_POINT ( 'NONE',  ( 73.07463722459043254, -55.71104259080762233, -34.59272409957256400 ) ) ;
#31121=DIRECTION ( 'NONE',  ( 0.9609149988134837450, -0.1028163501681639419, 0.2570431154366518145 ) ) ;
#31143=CARTESIAN_POINT ( 'NONE',  ( 70.19189222814998175, -51.68868231262963775, -33.87830190084585524 ) ) ;
#31145=ADVANCED_FACE ( 'NONE', ( #2059 ), #20508, .F. ) ;
#31152=CARTESIAN_POINT ( 'NONE',  ( 70.19189222814998175, -59.47700027789979060, -36.99360193826534271 ) ) ;
#31158=CIRCLE ( 'NONE', #17345, 2.999999999999999556 ) ;
#31177=DIRECTION ( 'NONE',  ( -0.000000000000000000, -0.9284778069183721172, -0.3713878862591650232 ) ) ;
#31182=EDGE_CURVE ( 'NONE', #44494, #44451, #23959, .T. ) ;
#31200=VERTEX_POINT ( 'NONE', #13245 ) ;
#31210=DIRECTION ( 'NONE',  ( 0.000000000000000000, 0.9284778069183720062, 0.3713878862591650232 ) ) ;
#31236=DIRECTION ( 'NONE',  ( -0.000000000000000000, -0.9284778069183721172, -0.3713878862591650232 ) ) ;
#31242=DIRECTION ( 'NONE',  ( -0.000000000000000000, -0.9284778069183718952, -0.3713878862591649677 ) ) ;
#31299=ORIENTED_EDGE ( 'NONE', *, *, #1047, .F. ) ;
#31300=VECTOR ( 'NONE', #37073, 1000.000000000000227 ) ;
#31306=CARTESIAN_POINT ( 'NONE',  ( 67.84197459855160162, -57.36860727972680252, -36.87942510454734446 ) ) ;
#31308=ORIENTED_EDGE ( 'NONE', *, *, #25940, .T. ) ;
#31326=CONICAL_SURFACE ( 'NONE', #28476, 2.999999999999999556, 0.9599310885968830309 ) ;
#31361=CIRCLE ( 'NONE', #39382, 2.445500000000004448 ) ;
#31362=CARTESIAN_POINT ( 'NONE',  ( 70.19189222814998175, -58.90901798090458641, -36.76641099935233825 ) ) ;
#31392=CARTESIAN_POINT ( 'NONE',  ( 70.19189222814998175, -65.04786711941001442, -39.22192925582032785 ) ) ;
#31433=ORIENTED_EDGE ( 'NONE', *, *, #21309, .F. ) ;
#31439=DIRECTION ( 'NONE',  ( -0.000000000000000000, -0.9284778069183721172, -0.3713878862591650232 ) ) ;
#31444=DIRECTION ( 'NONE',  ( 0.9609149988134837450, -0.1028163501681639419, 0.2570431154366518145 ) ) ;
#31482=CARTESIAN_POINT ( 'NONE',  ( 70.19189222814998175, -51.12070001563444066, -33.65111096193285078 ) ) ;
#31503=DIRECTION ( 'NONE',  ( 0.000000000000000000, 0.9284778069183720062, 0.3713878862591650232 ) ) ;
#31507=ORIENTED_EDGE ( 'NONE', *, *, #30017, .F. ) ;
#31508=CARTESIAN_POINT ( 'NONE',  ( 70.19189222814998175, -60.40547808481815650, -37.36498982452450690 ) ) ;
#31517=ORIENTED_EDGE ( 'NONE', *, *, #42098, .F. ) ;
#31520=VECTOR ( 'NONE', #134, 1000.000000000000227 ) ;
#31524=DIRECTION ( 'NONE',  ( 0.9609149988134837450, -0.1028163501681639419, 0.2570431154366518145 ) ) ;
#31534=AXIS2_PLACEMENT_3D ( 'NONE', #1832, #36711, #44035 ) ;
#31538=ADVANCED_FACE ( 'NONE', ( #21638 ), #37274, .T. ) ;
#31615=PLANE ( 'NONE',  #11005 ) ;
#31646=DIRECTION ( 'NONE',  ( -0.000000000000000000, -0.9284778069183721172, -0.3713878862591650232 ) ) ;
#31656=ORIENTED_EDGE ( 'NONE', *, *, #25043, .T. ) ;
#31666=DIRECTION ( 'NONE',  ( -0.2768435750659253847, -0.3568721902840677473, 0.8921882507333133150 ) ) ;
#31680=LINE ( 'NONE', #7289, #18653 ) ;
#31686=CYLINDRICAL_SURFACE ( 'NONE', #40177, 3.000000000000001776 ) ;
#31689=VERTEX_POINT ( 'NONE', #28714 ) ;
#31735=CIRCLE ( 'NONE', #23014, 2.445500000000004448 ) ;
#31802=EDGE_LOOP ( 'NONE', ( #23409, #12973, #24656, #34182, #19781 ) ) ;
#31868=EDGE_CURVE ( 'NONE', #8341, #33992, #42404, .T. ) ;
#31874=DIRECTION ( 'NONE',  ( 0.000000000000000000, 0.9284778069183720062, 0.3713878862591650232 ) ) ;
#31900=CARTESIAN_POINT ( 'NONE',  ( 70.19189222814998175, -52.97765562947117957, -34.39388673445118627 ) ) ;
#31906=DIRECTION ( 'NONE',  ( 0.9609149988134837450, -0.1028163501681639419, 0.2570431154366518145 ) ) ;
#31945=CARTESIAN_POINT ( 'NONE',  ( 70.19189222814998175, -60.04498257489500190, -37.22079287717834717 ) ) ;
#31959=ORIENTED_EDGE ( 'NONE', *, *, #5018, .F. ) ;
#31978=ORIENTED_EDGE ( 'NONE', *, *, #26998, .F. ) ;
#31986=LINE ( 'NONE', #10144, #4627 ) ;
#31993=DIRECTION ( 'NONE',  ( 0.7871354856660198740, 0.4483307682966886643, 0.4235767337848242442 ) ) ;
#32011=CIRCLE ( 'NONE', #42961, 3.000000000000001776 ) ;
#32026=AXIS2_PLACEMENT_3D ( 'NONE', #42169, #31439, #28260 ) ;
#32038=EDGE_CURVE ( 'NONE', #18777, #29125, #25729, .T. ) ;
#32080=DIRECTION ( 'NONE',  ( 0.9609149988134837450, -0.1028163501681639419, 0.2570431154366518145 ) ) ;
#32087=DIRECTION ( 'NONE',  ( 0.9609149988134837450, -0.1028163501681639419, 0.2570431154366518145 ) ) ;
#32100=AXIS2_PLACEMENT_3D ( 'NONE', #22257, #18616, #16094 ) ;
#32106=ORIENTED_EDGE ( 'NONE', *, *, #33402, .F. ) ;
#32120=ORIENTED_EDGE ( 'NONE', *, *, #5330, .F. ) ;
#32124=AXIS2_PLACEMENT_3D ( 'NONE', #15847, #22452, #40696 ) ;
#32153=DIRECTION ( 'NONE',  ( -0.000000000000000000, -0.9284778069183718952, -0.3713878862591649677 ) ) ;
#32167=FACE_OUTER_BOUND ( 'NONE', #28058, .T. ) ;
#32172=DIRECTION ( 'NONE',  ( 0.7871354856660167654, -0.6167752151498625546, -0.002461946824136807422 ) ) ;
#32174=DIRECTION ( 'NONE',  ( -0.9609149988134834119, 0.1028163501681648995, -0.2570431154366529802 ) ) ;
#32189=LINE ( 'NONE', #26934, #43362 ) ;
#32198=VERTEX_POINT ( 'NONE', #28480 ) ;
#32204=ORIENTED_EDGE ( 'NONE', *, *, #33337, .F. ) ;
#32240=CYLINDRICAL_SURFACE ( 'NONE', #6601, 5.000000000000002665 ) ;
#32249=ADVANCED_FACE ( 'NONE', ( #871 ), #17664, .T. ) ;
#32251=ADVANCED_FACE ( 'NONE', ( #35515 ), #35107, .T. ) ;
#32254=DIRECTION ( 'NONE',  ( 0.9609149988134837450, -0.1028163501681639419, 0.2570431154366518145 ) ) ;
#32259=AXIS2_PLACEMENT_3D ( 'NONE', #15897, #23189, #44173 ) ;
#32300=DIRECTION ( 'NONE',  ( -0.000000000000000000, -0.9284778069183721172, -0.3713878862591650232 ) ) ;
#32308=ADVANCED_FACE ( 'NONE', ( #8209 ), #4778, .T. ) ;
#32317=ORIENTED_EDGE ( 'NONE', *, *, #4709, .T. ) ;
#32341=ORIENTED_EDGE ( 'NONE', *, *, #22250, .F. ) ;
#32346=FACE_OUTER_BOUND ( 'NONE', #15465, .T. ) ;
#32364=EDGE_LOOP ( 'NONE', ( #11166, #35267, #20264, #3391, #6886 ) ) ;
#32365=EDGE_CURVE ( 'NONE', #26037, #11292, #13320, .T. ) ;
#32369=CIRCLE ( 'NONE', #41130, 2.999999999999999556 ) ;
#32402=CIRCLE ( 'NONE', #6182, 2.999999999999999556 ) ;
#32414=EDGE_CURVE ( 'NONE', #23460, #15244, #43315, .T. ) ;
#32423=ORIENTED_EDGE ( 'NONE', *, *, #8269, .F. ) ;
#32438=AXIS2_PLACEMENT_3D ( 'NONE', #3278, #44346, #16755 ) ;
#32440=DIRECTION ( 'NONE',  ( -0.2768435750659241079, -0.3568721902840695792, 0.8921882507333129819 ) ) ;
#32470=ORIENTED_EDGE ( 'NONE', *, *, #23388, .T. ) ;
#32476=CARTESIAN_POINT ( 'NONE',  ( 69.36136150295220659, -58.33016572499207797, -33.43006446620090344 ) ) ;
#32495=DIRECTION ( 'NONE',  ( -0.000000000000000000, -0.9284778069183721172, -0.3713878862591650232 ) ) ;
#32529=DIRECTION ( 'NONE',  ( 0.9609149988134837450, -0.1028163501681639419, 0.2570431154366518145 ) ) ;
#32530=VERTEX_POINT ( 'NONE', #5898 ) ;
#32532=CIRCLE ( 'NONE', #36918, 2.445500000000004448 ) ;
#32539=CYLINDRICAL_SURFACE ( 'NONE', #12185, 3.000000000000001776 ) ;
#32547=VECTOR ( 'NONE', #5396, 1000.000000000000227 ) ;
#32553=DIRECTION ( 'NONE',  ( -0.000000000000000000, -0.9284778069183721172, -0.3713878862591650232 ) ) ;
#32557=ORIENTED_EDGE ( 'NONE', *, *, #6632, .F. ) ;
#32562=DIRECTION ( 'NONE',  ( -0.000000000000000000, -0.9284778069183721172, -0.3713878862591650232 ) ) ;
#32568=CIRCLE ( 'NONE', #43523, 2.999999999999999556 ) ;
#32592=LINE ( 'NONE', #5676, #26696 ) ;
#32596=( GEOMETRIC_REPRESENTATION_CONTEXT ( 3 ) GLOBAL_UNCERTAINTY_ASSIGNED_CONTEXT ( ( #8251 ) ) GLOBAL_UNIT_ASSIGNED_CONTEXT ( ( #25752, #39658, #12749 ) ) REPRESENTATION_CONTEXT ( 'NONE', 'WORKASPACE' ) );
#32598=CARTESIAN_POINT ( 'NONE',  ( 72.54180985774836188, -56.94300424148091366, -35.25083934068751290 ) ) ;
#32631=CARTESIAN_POINT ( 'NONE',  ( 71.02242295334774269, -51.54654354869580857, -36.92625453930496349 ) ) ;
#32639=EDGE_LOOP ( 'NONE', ( #38922, #6550, #30426, #15805, #41863, #8777 ) ) ;
#32698=DIRECTION ( 'NONE',  ( 0.9609149988134843001, -0.1028163501681632064, 0.2570431154366505933 ) ) ;
#32735=DIRECTION ( 'NONE',  ( -0.7871354856660202071, 0.6167752151498580027, 0.002461946824133919541 ) ) ;
#32736=ORIENTED_EDGE ( 'NONE', *, *, #40464, .T. ) ;
#32737=DIRECTION ( 'NONE',  ( 0.9609149988134843001, -0.1028163501681632064, 0.2570431154366505933 ) ) ;
#32749=AXIS2_PLACEMENT_3D ( 'NONE', #12837, #36748, #19893 ) ;
#32762=CONICAL_SURFACE ( 'NONE', #5108, 2.445500000000004448, 0.9599310885968757034 ) ;
#32774=CARTESIAN_POINT ( 'NONE',  ( 72.54180985774836188, -55.08604862764417476, -34.50806356816917742 ) ) ;
#32785=EDGE_CURVE ( 'NONE', #25810, #12184, #7246, .T. ) ;
#32798=ORIENTED_EDGE ( 'NONE', *, *, #11649, .F. ) ;
#32809=LINE ( 'NONE', #18918, #30303 ) ;
#32840=EDGE_CURVE ( 'NONE', #39890, #14756, #38041, .T. ) ;
#32853=DIRECTION ( 'NONE',  ( 0.9609149988134837450, -0.1028163501681639419, 0.2570431154366518145 ) ) ;
#32855=VERTEX_POINT ( 'NONE', #20278 ) ;
#32861=VERTEX_POINT ( 'NONE', #9056 ) ;
#32862=ORIENTED_EDGE ( 'NONE', *, *, #3022, .T. ) ;
#32876=VERTEX_POINT ( 'NONE', #22956 ) ;
#32915=DIRECTION ( 'NONE',  ( 0.9609149988134837450, -0.1028163501681639419, 0.2570431154366518145 ) ) ;
#32930=AXIS2_PLACEMENT_3D ( 'NONE', #42384, #11148, #25052 ) ;
#32942=DIRECTION ( 'NONE',  ( 0.9609149988134839671, -0.1028163501681660097, 0.2570431154366504822 ) ) ;
#32981=VECTOR ( 'NONE', #18951, 1000.000000000000114 ) ;
#32998=CONICAL_SURFACE ( 'NONE', #40317, 2.999999999999999556, 0.9599310885968830309 ) ;
#33002=VERTEX_POINT ( 'NONE', #8603 ) ;
#33014=DIRECTION ( 'NONE',  ( 0.7202110682883375858, 0.2576522076061144029, -0.6441361323747234469 ) ) ;
#33021=VERTEX_POINT ( 'NONE', #22504 ) ;
#33026=AXIS2_PLACEMENT_3D ( 'NONE', #42319, #14723, #17695 ) ;
#33034=DIRECTION ( 'NONE',  ( 0.9609149988134837450, -0.1028163501681639419, 0.2570431154366518145 ) ) ;
#33042=CIRCLE ( 'NONE', #38881, 2.999999999999999556 ) ;
#33078=VECTOR ( 'NONE', #39454, 1000.000000000000227 ) ;
#33082=VERTEX_POINT ( 'NONE', #10412 ) ;
#33087=EDGE_CURVE ( 'NONE', #26262, #18481, #22055, .T. ) ;
#33088=ORIENTED_EDGE ( 'NONE', *, *, #495, .F. ) ;
#33091=EDGE_CURVE ( 'NONE', #20113, #34097, #3153, .T. ) ;
#33092=CARTESIAN_POINT ( 'NONE',  ( 70.19189222814998175, -59.11650476797663600, -36.84940499091918298 ) ) ;
#33100=EDGE_CURVE ( 'NONE', #31200, #40221, #17036, .T. ) ;
#33101=LINE ( 'NONE', #23557, #37301 ) ;
#33117=CIRCLE ( 'NONE', #9852, 4.999999999999998224 ) ;
#33138=DIRECTION ( 'NONE',  ( 0.7871354856660167654, -0.6167752151498625546, -0.002461946824136807422 ) ) ;
#33145=CARTESIAN_POINT ( 'NONE',  ( 70.19189222814998175, -59.11650476797663600, -36.84940499091918298 ) ) ;
#33155=ADVANCED_FACE ( 'NONE', ( #37990 ), #6535, .T. ) ;
#33156=CARTESIAN_POINT ( 'NONE',  ( 70.19189222814998175, -60.04498257489500190, -37.22079287717834717 ) ) ;
#33178=EDGE_CURVE ( 'NONE', #34283, #6949, #38424, .T. ) ;
#33183=CIRCLE ( 'NONE', #15725, 2.999999999999999556 ) ;
#33201=CIRCLE ( 'NONE', #13579, 2.541999999999999371 ) ;
#33236=VERTEX_POINT ( 'NONE', #32476 ) ;
#33272=VECTOR ( 'NONE', #20236, 1000.000000000000227 ) ;
#33302=EDGE_LOOP ( 'NONE', ( #9266, #25767, #10542, #40022 ) ) ;
#33309=ORIENTED_EDGE ( 'NONE', *, *, #22838, .F. ) ;
#33331=CARTESIAN_POINT ( 'NONE',  ( 70.19189222814998175, -58.90901798090458641, -36.76641099935233825 ) ) ;
#33337=EDGE_CURVE ( 'NONE', #38926, #1783, #41723, .T. ) ;
#33345=FACE_OUTER_BOUND ( 'NONE', #23647, .T. ) ;
#33350=EDGE_CURVE ( 'NONE', #43627, #22284, #28632, .T. ) ;
#33369=DIRECTION ( 'NONE',  ( 0.9609149988134843001, -0.1028163501681632064, 0.2570431154366505933 ) ) ;
#33372=DIRECTION ( 'NONE',  ( 0.9609149988134837450, -0.1028163501681639419, 0.2570431154366518145 ) ) ;
#33402=EDGE_CURVE ( 'NONE', #19524, #22169, #22225, .T. ) ;
#33407=EDGE_LOOP ( 'NONE', ( #40505, #8567, #26049, #22615, #36971 ) ) ;
#33414=ORIENTED_EDGE ( 'NONE', *, *, #5784, .F. ) ;
#33415=CIRCLE ( 'NONE', #17434, 2.445500000000004448 ) ;
#33419=LINE ( 'NONE', #12940, #38576 ) ;
#33427=DIRECTION ( 'NONE',  ( -0.000000000000000000, -0.9284778069183718952, -0.3713878862591649677 ) ) ;
#33459=SHAPE_REPRESENTATION_RELATIONSHIP ( 'NONE' , 'NONE' ,  #10805, #16689 ) ;
#33476=CIRCLE ( 'NONE', #36386, 2.999999999999999556 ) ;
#33477=DIRECTION ( 'NONE',  ( -0.000000000000000000, -0.9284778069183718952, -0.3713878862591649677 ) ) ;
#33483=DIRECTION ( 'NONE',  ( -0.9609149988134837450, 0.1028163501681639419, -0.2570431154366518145 ) ) ;
#33484=AXIS2_PLACEMENT_3D ( 'NONE', #11663, #25572, #1388 ) ;
#33500=ORIENTED_EDGE ( 'NONE', *, *, #12796, .T. ) ;
#33524=ORIENTED_EDGE ( 'NONE', *, *, #26991, .F. ) ;
#33531=EDGE_LOOP ( 'NONE', ( #12598, #2690, #35951, #43266, #32106 ) ) ;
#33537=CARTESIAN_POINT ( 'NONE',  ( 69.36136150295220659, -101.1685209014307674, -50.56525720990386219 ) ) ;
#33556=VECTOR ( 'NONE', #30810, 1000.000000000000114 ) ;
#33581=AXIS2_PLACEMENT_3D ( 'NONE', #44348, #24272, #13108 ) ;
#33607=FACE_OUTER_BOUND ( 'NONE', #23183, .T. ) ;
#33630=ADVANCED_FACE ( 'NONE', ( #18806 ), #33693, .T. ) ;
#33632=VERTEX_POINT ( 'NONE', #30198 ) ;
#33641=AXIS2_PLACEMENT_3D ( 'NONE', #3248, #31503, #14184 ) ;
#33689=( GEOMETRIC_REPRESENTATION_CONTEXT ( 3 ) GLOBAL_UNCERTAINTY_ASSIGNED_CONTEXT ( ( #41585 ) ) GLOBAL_UNIT_ASSIGNED_CONTEXT ( ( #23464, #9782, #30746 ) ) REPRESENTATION_CONTEXT ( 'NONE', 'WORKASPACE' ) );
#33693=CONICAL_SURFACE ( 'NONE', #27896, 2.999999999999999556, 0.9599310885968830309 ) ;
#33698=CARTESIAN_POINT ( 'NONE',  ( 70.89841814381148311, -68.89136543047671069, -37.69090763720760151 ) ) ;
#33719=DIRECTION ( 'NONE',  ( 0.000000000000000000, 0.9284778069183720062, 0.3713878862591650232 ) ) ;
#33744=VECTOR ( 'NONE', #32735, 1000.000000000000114 ) ;
#33755=EDGE_CURVE ( 'NONE', #32861, #20113, #24255, .T. ) ;
#33769=ORIENTED_EDGE ( 'NONE', *, *, #2761, .T. ) ;
#33800=ORIENTED_EDGE ( 'NONE', *, *, #37354, .F. ) ;
#33811=ORIENTED_EDGE ( 'NONE', *, *, #9220, .F. ) ;
#33817=ORIENTED_EDGE ( 'NONE', *, *, #6423, .T. ) ;
#33818=DIRECTION ( 'NONE',  ( -0.9609149988134837450, 0.1028163501681639419, -0.2570431154366518145 ) ) ;
#33824=CARTESIAN_POINT ( 'NONE',  ( 70.19189222814998175, -61.33395589173652951, -37.73637771078367109 ) ) ;
#33842=PLANE ( 'NONE',  #1772 ) ;
#33871=ORIENTED_EDGE ( 'NONE', *, *, #1919, .F. ) ;
#33873=CIRCLE ( 'NONE', #20777, 2.999999999999999556 ) ;
#33936=VECTOR ( 'NONE', #27912, 1000.000000000000227 ) ;
#33966=DIRECTION ( 'NONE',  ( 0.9609149988134843001, -0.1028163501681632064, 0.2570431154366505933 ) ) ;
#33970=DIRECTION ( 'NONE',  ( -0.7871354856660162103, -0.4483307682966942709, -0.4235767337848251879 ) ) ;
#33981=DIRECTION ( 'NONE',  ( -0.2768435750659241079, -0.3568721902840695792, 0.8921882507333129819 ) ) ;
#33992=VERTEX_POINT ( 'NONE', #7220 ) ;
#33998=VECTOR ( 'NONE', #16556, 1000.000000000000114 ) ;
#34033=DIRECTION ( 'NONE',  ( -0.000000000000000000, -0.9284778069183718952, -0.3713878862591649677 ) ) ;
#34052=EDGE_CURVE ( 'NONE', #31689, #37171, #8796, .T. ) ;
#34086=DIRECTION ( 'NONE',  ( -0.000000000000000000, -0.9284778069183721172, -0.3713878862591650232 ) ) ;
#34097=VERTEX_POINT ( 'NONE', #5590 ) ;
#34116=FACE_OUTER_BOUND ( 'NONE', #17479, .T. ) ;
#34119=DIRECTION ( 'NONE',  ( -0.000000000000000000, -0.9284778069183720062, -0.3713878862591650232 ) ) ;
#34121=FACE_OUTER_BOUND ( 'NONE', #38059, .T. ) ;
#34131=DIRECTION ( 'NONE',  ( 0.9609149988134843001, -0.1028163501681632064, 0.2570431154366505933 ) ) ;
#34150=ORIENTED_EDGE ( 'NONE', *, *, #6053, .T. ) ;
#34182=ORIENTED_EDGE ( 'NONE', *, *, #28698, .F. ) ;
#34190=EDGE_LOOP ( 'NONE', ( #39392, #27112, #42249, #38468, #23763, #35955 ) ) ;
#34215=VERTEX_POINT ( 'NONE', #19060 ) ;
#34223=CIRCLE ( 'NONE', #39337, 2.999999999999999556 ) ;
#34232=FACE_OUTER_BOUND ( 'NONE', #28171, .T. ) ;
#34239=EDGE_LOOP ( 'NONE', ( #37466, #2686, #3915, #24606, #1303 ) ) ;
#34242=LINE ( 'NONE', #7104, #23489 ) ;
#34274=VERTEX_POINT ( 'NONE', #36821 ) ;
#34283=VERTEX_POINT ( 'NONE', #18833 ) ;
#34288=AXIS2_PLACEMENT_3D ( 'NONE', #8664, #5911, #33034 ) ;
#34307=CARTESIAN_POINT ( 'NONE',  ( 70.19189222814998175, -100.0979043305785581, -53.24182196210380624 ) ) ;
#34309=DIRECTION ( 'NONE',  ( 0.9609149988134843001, -0.1028163501681632064, 0.2570431154366505933 ) ) ;
#34327=ORIENTED_EDGE ( 'NONE', *, *, #43419, .F. ) ;
#34334=ORIENTED_EDGE ( 'NONE', *, *, #18597, .T. ) ;
#34335=DIRECTION ( 'NONE',  ( 0.9609149988134837450, -0.1028163501681639419, 0.2570431154366518145 ) ) ;
#34346=DIRECTION ( 'NONE',  ( 0.9609149988134837450, -0.1028163501681639419, 0.2570431154366518145 ) ) ;
#34368=EDGE_LOOP ( 'NONE', ( #38096, #38043, #41066, #37126, #41702 ) ) ;
#34370=ORIENTED_EDGE ( 'NONE', *, *, #36438, .T. ) ;
#34428=AXIS2_PLACEMENT_3D ( 'NONE', #37400, #5935, #2516 ) ;
#34430=CONICAL_SURFACE ( 'NONE', #43169, 2.445500000000005336, 0.9599310885968757034 ) ;
#34473=EDGE_LOOP ( 'NONE', ( #5246, #27145, #20280, #14368, #17432 ) ) ;
#34491=EDGE_CURVE ( 'NONE', #1665, #2964, #16325, .T. ) ;
#34504=EDGE_CURVE ( 'NONE', #17518, #29144, #44214, .T. ) ;
#34508=EDGE_CURVE ( 'NONE', #36514, #25917, #2396, .T. ) ;
#34511=DIRECTION ( 'NONE',  ( -0.7871354856660162103, -0.4483307682966942709, -0.4235767337848251879 ) ) ;
#34523=AXIS2_PLACEMENT_3D ( 'NONE', #23942, #41495, #37821 ) ;
#34527=CARTESIAN_POINT ( 'NONE',  ( 67.37136766119182596, -67.53150897494617766, -41.09057840265009531 ) ) ;
#34529=CARTESIAN_POINT ( 'NONE',  ( 70.19189222814998175, -60.97346038181336070, -37.59218076343751136 ) ) ;
#34551=AXIS2_PLACEMENT_3D ( 'NONE', #31152, #34776, #3559 ) ;
#34564=PLANE ( 'NONE',  #11390 ) ;
#34569=EDGE_CURVE ( 'NONE', #16121, #279, #19966, .T. ) ;
#34580=CARTESIAN_POINT ( 'NONE',  ( 70.89841814381148311, -71.67679885123182260, -38.80507129598510119 ) ) ;
#34583=CARTESIAN_POINT ( 'NONE',  ( 69.36136150295220659, -52.55181209640981166, -31.11874315707907357 ) ) ;
#34628=AXIS2_PLACEMENT_3D ( 'NONE', #3082, #17442, #34309 ) ;
#34633=PLANE ( 'NONE',  #39524 ) ;
#34648=AXIS2_PLACEMENT_3D ( 'NONE', #10140, #2827, #19940 ) ;
#34667=AXIS2_PLACEMENT_3D ( 'NONE', #40818, #44460, #27127 ) ;
#34682=ORIENTED_EDGE ( 'NONE', *, *, #20144, .T. ) ;
#34703=VECTOR ( 'NONE', #13362, 1000.000000000000227 ) ;
#34709=AXIS2_PLACEMENT_3D ( 'NONE', #13668, #20510, #40809 ) ;
#34714=LINE ( 'NONE', #31306, #26053 ) ;
#34717=CARTESIAN_POINT ( 'NONE',  ( 70.19189222814998175, -53.33815113939435548, -34.53808368179734600 ) ) ;
#34720=CIRCLE ( 'NONE', #4888, 2.999999999999999556 ) ;
#34725=VERTEX_POINT ( 'NONE', #43188 ) ;
#34754=ORIENTED_EDGE ( 'NONE', *, *, #15840, .T. ) ;
#34758=AXIS2_PLACEMENT_3D ( 'NONE', #2839, #20188, #6725 ) ;
#34770=DIRECTION ( 'NONE',  ( -0.000000000000000000, -0.9284778069183721172, -0.3713878862591650232 ) ) ;
#34776=DIRECTION ( 'NONE',  ( -0.000000000000000000, -0.9284778069183720062, -0.3713878862591650232 ) ) ;
#34780=EDGE_CURVE ( 'NONE', #42481, #19894, #10120, .T. ) ;
#34827=CARTESIAN_POINT ( 'NONE',  ( 70.19189222814998175, -56.69156685714467159, -35.87943827948784303 ) ) ;
#34835=ORIENTED_EDGE ( 'NONE', *, *, #30870, .T. ) ;
#34873=AXIS2_PLACEMENT_3D ( 'NONE', #17500, #32300, #11566 ) ;
#34887=VERTEX_POINT ( 'NONE', #5700 ) ;
#34915=CARTESIAN_POINT ( 'NONE',  ( 67.30914723170953096, -59.73653352439050934, -37.99192222348830938 ) ) ;
#34918=CARTESIAN_POINT ( 'NONE',  ( 67.72463061902256243, -68.06054142010196983, -39.76798576395498941 ) ) ;
#34942=VECTOR ( 'NONE', #32174, 1000.000000000000114 ) ;
#34968=DIRECTION ( 'NONE',  ( 0.7871354856660167654, -0.6167752151498625546, -0.002461946824136807422 ) ) ;
#35006=VECTOR ( 'NONE', #29954, 1000.000000000000227 ) ;
#35040=AXIS2_PLACEMENT_3D ( 'NONE', #23325, #37682, #6680 ) ;
#35044=CARTESIAN_POINT ( 'NONE',  ( 69.36136150295220659, -101.1685209014307674, -50.56525720990386219 ) ) ;
#35046=CARTESIAN_POINT ( 'NONE',  ( 70.19189222814998175, -61.69445140165969121, -37.88057465812982372 ) ) ;
#35066=ORIENTED_EDGE ( 'NONE', *, *, #26137, .F. ) ;
#35091=ORIENTED_EDGE ( 'NONE', *, *, #10044, .F. ) ;
#35107=CONICAL_SURFACE ( 'NONE', #43147, 2.445500000000004448, 0.9599310885968757034 ) ;
#35113=DIRECTION ( 'NONE',  ( -0.7871354856660202071, 0.6167752151498580027, 0.002461946824133919541 ) ) ;
#35126=ADVANCED_FACE ( 'NONE', ( #6313 ), #42766, .T. ) ;
#35131=VECTOR ( 'NONE', #33014, 1000.000000000000114 ) ;
#35134=VERTEX_POINT ( 'NONE', #26388 ) ;
#35170=CARTESIAN_POINT ( 'NONE',  ( 70.19189222814998175, -53.54563792646638376, -34.62107767336419073 ) ) ;
#35187=STYLED_ITEM ( 'NONE', ( #30292 ), #16689 ) ;
#35202=VERTEX_POINT ( 'NONE', #23197 ) ;
#35216=DIRECTION ( 'NONE',  ( -0.000000000000000000, -0.9284778069183721172, -0.3713878862591650232 ) ) ;
#35221=CARTESIAN_POINT ( 'NONE',  ( 70.19189222814998175, -100.0979043305785581, -53.24182196210380624 ) ) ;
#35242=FACE_OUTER_BOUND ( 'NONE', #27508, .T. ) ;
#35267=ORIENTED_EDGE ( 'NONE', *, *, #4967, .T. ) ;
#35273=CARTESIAN_POINT ( 'NONE',  ( 67.84197459855160162, -55.51165166589005651, -36.13664933202900897 ) ) ;
#35277=VECTOR ( 'NONE', #23482, 1000.000000000000227 ) ;
#35278=CARTESIAN_POINT ( 'NONE',  ( 70.19189222814998175, -56.33107134722149567, -35.73524133214168330 ) ) ;
#35291=CARTESIAN_POINT ( 'NONE',  ( 70.19189222814998175, -52.61716011954800365, -34.24968978710501943 ) ) ;
#35294=VERTEX_POINT ( 'NONE', #6079 ) ;
#35303=ORIENTED_EDGE ( 'NONE', *, *, #22638, .F. ) ;
#35323=ADVANCED_FACE ( 'NONE', ( #30032 ), #10555, .T. ) ;
#35324=ADVANCED_FACE ( 'NONE', ( #27299 ), #41875, .T. ) ;
#35345=CARTESIAN_POINT ( 'NONE',  ( 69.36136150295220659, -62.04407695266556289, -34.91561601123756731 ) ) ;
#35346=AXIS2_PLACEMENT_3D ( 'NONE', #28528, #4108, #42210 ) ;
#35372=ORIENTED_EDGE ( 'NONE', *, *, #35560, .F. ) ;
#35389=CARTESIAN_POINT ( 'NONE',  ( 70.19189222814998175, -52.97765562947117957, -34.39388673445118627 ) ) ;
#35392=ORIENTED_EDGE ( 'NONE', *, *, #32414, .F. ) ;
#35418=DIRECTION ( 'NONE',  ( 0.9609149988134837450, -0.1028163501681639419, 0.2570431154366518145 ) ) ;
#35436=ORIENTED_EDGE ( 'NONE', *, *, #23419, .F. ) ;
#35482=DIRECTION ( 'NONE',  ( -0.000000000000000000, -0.9284778069183721172, -0.3713878862591650232 ) ) ;
#35502=CIRCLE ( 'NONE', #27528, 0.3000000000000022093 ) ;
#35515=FACE_OUTER_BOUND ( 'NONE', #41576, .T. ) ;
#35526=CARTESIAN_POINT ( 'NONE',  ( 70.19189222814998175, -53.90613343638955968, -34.76527462071035046 ) ) ;
#35545=FACE_OUTER_BOUND ( 'NONE', #36655, .T. ) ;
#35560=EDGE_CURVE ( 'NONE', #4821, #32198, #25806, .T. ) ;
#35573=ORIENTED_EDGE ( 'NONE', *, *, #21018, .T. ) ;
#35623=EDGE_CURVE ( 'NONE', #35134, #279, #36009, .T. ) ;
#35628=DIRECTION ( 'NONE',  ( 0.2768435750659241079, 0.3568721902840695792, -0.8921882507333129819 ) ) ;
#35636=VERTEX_POINT ( 'NONE', #7205 ) ;
#35646=CARTESIAN_POINT ( 'NONE',  ( 70.19189222814998175, -57.98054017398621340, -36.39502311309316696 ) ) ;
#35670=CIRCLE ( 'NONE', #22560, 2.445500000000004448 ) ;
#35671=LINE ( 'NONE', #352, #4143 ) ;
#35729=CARTESIAN_POINT ( 'NONE',  ( 68.07789357685331311, -68.58957386525776201, -38.44539312525987640 ) ) ;
#35730=CARTESIAN_POINT ( 'NONE',  ( 70.19189222814998175, -52.40967333247598248, -34.16669579553818181 ) ) ;
#35766=CARTESIAN_POINT ( 'NONE',  ( 71.02242295334774269, -57.83840141005237712, -39.44297575155226809 ) ) ;
#35788=DIRECTION ( 'NONE',  ( -0.2768435750659241079, -0.3568721902840695792, 0.8921882507333129819 ) ) ;
#35800=VERTEX_POINT ( 'NONE', #13119 ) ;
#35828=DIRECTION ( 'NONE',  ( -0.000000000000000000, -0.9284778069183721172, -0.3713878862591650232 ) ) ;
#35830=ORIENTED_EDGE ( 'NONE', *, *, #17762, .F. ) ;
#35854=LINE ( 'NONE', #8963, #9294 ) ;
#35869=AXIS2_PLACEMENT_3D ( 'NONE', #24749, #35216, #25207 ) ;
#35897=ADVANCED_FACE ( 'NONE', ( #33607 ), #33842, .T. ) ;
#35901=CIRCLE ( 'NONE', #12633, 2.999999999999999556 ) ;
#35906=DIRECTION ( 'NONE',  ( 0.9609149988134837450, -0.1028163501681639419, 0.2570431154366518145 ) ) ;
#35939=ORIENTED_EDGE ( 'NONE', *, *, #41607, .T. ) ;
#35951=ORIENTED_EDGE ( 'NONE', *, *, #179, .T. ) ;
#35955=ORIENTED_EDGE ( 'NONE', *, *, #14423, .F. ) ;
#35956=CYLINDRICAL_SURFACE ( 'NONE', #16774, 3.000000000000001776 ) ;
#35964=CARTESIAN_POINT ( 'NONE',  ( 67.84197459855160162, -49.94078482437982558, -33.90832201447402383 ) ) ;
#35966=LINE ( 'NONE', #26393, #20162 ) ;
#35989=LINE ( 'NONE', #14582, #43051 ) ;
#35994=DIRECTION ( 'NONE',  ( -0.7871354856660162103, -0.4483307682966942709, -0.4235767337848251879 ) ) ;
#36009=CIRCLE ( 'NONE', #41866, 2.999999999999999556 ) ;
#36037=DIRECTION ( 'NONE',  ( -0.2768435750659239414, -0.3568721902840664151, 0.8921882507333142032 ) ) ;
#36039=FACE_OUTER_BOUND ( 'NONE', #7302, .T. ) ;
#36045=ORIENTED_EDGE ( 'NONE', *, *, #20015, .F. ) ;
#36056=CARTESIAN_POINT ( 'NONE',  ( 70.19189222814998175, -57.05206236706784040, -36.02363522683400276 ) ) ;
#36058=EDGE_LOOP ( 'NONE', ( #23278, #5280, #128, #33769, #16573, #27555 ) ) ;
#36073=AXIS2_PLACEMENT_3D ( 'NONE', #9863, #10311, #24427 ) ;
#36081=CONICAL_SURFACE ( 'NONE', #12810, 2.445500000000004448, 0.9599310885968757034 ) ;
#36123=DIRECTION ( 'NONE',  ( -0.000000000000000000, -0.9284778069183721172, -0.3713878862591650232 ) ) ;
#36132=ADVANCED_FACE ( 'NONE', ( #42038 ), #36725, .T. ) ;
#36164=CARTESIAN_POINT ( 'NONE',  ( 69.36136150295220659, -60.90811235867516160, -34.46123413341155839 ) ) ;
#36176=VERTEX_POINT ( 'NONE', #22398 ) ;
#36177=AXIS2_PLACEMENT_3D ( 'NONE', #37539, #2428, #23194 ) ;
#36207=DIRECTION ( 'NONE',  ( -0.000000000000000000, -0.9284778069183721172, -0.3713878862591650232 ) ) ;
#36212=DIRECTION ( 'NONE',  ( 0.9609149988134837450, -0.1028163501681639419, 0.2570431154366518145 ) ) ;
#36226=ORIENTED_EDGE ( 'NONE', *, *, #25199, .F. ) ;
#36258=AXIS2_PLACEMENT_3D ( 'NONE', #1113, #3852, #17997 ) ;
#36263=DIRECTION ( 'NONE',  ( -0.000000000000000000, -0.9284778069183721172, -0.3713878862591650232 ) ) ;
#36270=ORIENTED_EDGE ( 'NONE', *, *, #15945, .F. ) ;
#36279=VERTEX_POINT ( 'NONE', #40635 ) ;
#36322=EDGE_CURVE ( 'NONE', #27364, #18078, #32369, .T. ) ;
#36346=AXIS2_PLACEMENT_3D ( 'NONE', #5529, #25840, #36539 ) ;
#36361=ORIENTED_EDGE ( 'NONE', *, *, #26999, .T. ) ;
#36386=AXIS2_PLACEMENT_3D ( 'NONE', #12059, #32562, #39867 ) ;
#36394=CARTESIAN_POINT ( 'NONE',  ( 70.19189222814998175, -100.0979043305785581, -53.24182196210380624 ) ) ;
#36397=AXIS2_PLACEMENT_3D ( 'NONE', #17913, #28405, #14269 ) ;
#36431=ORIENTED_EDGE ( 'NONE', *, *, #25758, .F. ) ;
#36438=EDGE_CURVE ( 'NONE', #11921, #10287, #32402, .T. ) ;
#36488=LINE ( 'NONE', #41457, #8815 ) ;
#36497=VECTOR ( 'NONE', #27310, 1000.000000000000227 ) ;
#36514=VERTEX_POINT ( 'NONE', #16468 ) ;
#36529=DIRECTION ( 'NONE',  ( 0.9609149988134843001, -0.1028163501681632064, 0.2570431154366505933 ) ) ;
#36539=DIRECTION ( 'NONE',  ( 0.9609149988134837450, -0.1028163501681639419, 0.2570431154366518145 ) ) ;
#36562=VERTEX_POINT ( 'NONE', #6432 ) ;
#36564=EDGE_CURVE ( 'NONE', #18777, #35294, #12763, .T. ) ;
#36570=CARTESIAN_POINT ( 'NONE',  ( 68.07789357685331311, -71.37500728601287392, -39.55955678403736897 ) ) ;
#36579=EDGE_LOOP ( 'NONE', ( #9958, #41224, #6484 ) ) ;
#36627=CARTESIAN_POINT ( 'NONE',  ( 67.30914723170953096, -54.88665770272660183, -36.05198880062562949 ) ) ;
#36637=AXIS2_PLACEMENT_3D ( 'NONE', #22317, #14575, #36212 ) ;
#36655=EDGE_LOOP ( 'NONE', ( #24182, #12386, #10721, #17555 ) ) ;
#36711=DIRECTION ( 'NONE',  ( -0.000000000000000000, -0.9284778069183721172, -0.3713878862591650232 ) ) ;
#36718=ADVANCED_FACE ( 'NONE', ( #21894 ), #25327, .T. ) ;
#36725=CONICAL_SURFACE ( 'NONE', #1068, 2.445500000000004448, 0.9599310885968757034 ) ;
#36732=CIRCLE ( 'NONE', #25099, 2.999999999999999556 ) ;
#36743=DIRECTION ( 'NONE',  ( -0.000000000000000000, -0.9284778069183718952, -0.3713878862591649677 ) ) ;
#36748=DIRECTION ( 'NONE',  ( -0.000000000000000000, -0.9284778069183721172, -0.3713878862591650232 ) ) ;
#36749=ORIENTED_EDGE ( 'NONE', *, *, #33337, .T. ) ;
#36751=ADVANCED_FACE ( 'NONE', ( #8442 ), #28776, .T. ) ;
#36753=AXIS2_PLACEMENT_3D ( 'NONE', #24374, #18195, #7930 ) ;
#36765=CIRCLE ( 'NONE', #4718, 2.999999999999999556 ) ;
#36787=VECTOR ( 'NONE', #25939, 1000.000000000000000 ) ;
#36796=CARTESIAN_POINT ( 'NONE',  ( 73.07463722459043254, -62.93137825908255678, -37.48083319807903280 ) ) ;
#36821=CARTESIAN_POINT ( 'NONE',  ( 73.07463722459043254, -58.28898922449070596, -35.62389376678321184 ) ) ;
#36851=DIRECTION ( 'NONE',  ( 0.000000000000000000, 0.9284778069183720062, 0.3713878862591650232 ) ) ;
#36856=DIRECTION ( 'NONE',  ( 0.9609149988134843001, -0.1028163501681632064, 0.2570431154366505933 ) ) ;
#36857=CIRCLE ( 'NONE', #26660, 2.999999999999999556 ) ;
#36873=DIRECTION ( 'NONE',  ( 0.9609149988134837450, -0.1028163501681639419, 0.2570431154366518145 ) ) ;
#36882=ORIENTED_EDGE ( 'NONE', *, *, #40516, .F. ) ;
#36886=ORIENTED_EDGE ( 'NONE', *, *, #17508, .T. ) ;
#36891=FACE_OUTER_BOUND ( 'NONE', #3705, .T. ) ;
#36894=CIRCLE ( 'NONE', #17963, 2.999999999999999556 ) ;
#36910=FACE_OUTER_BOUND ( 'NONE', #27256, .T. ) ;
#36918=AXIS2_PLACEMENT_3D ( 'NONE', #28414, #24331, #39117 ) ;
#36936=CARTESIAN_POINT ( 'NONE',  ( 67.30914723170953096, -56.95110010363538322, -36.87775856471080260 ) ) ;
#36971=ORIENTED_EDGE ( 'NONE', *, *, #3140, .F. ) ;
#36995=DIRECTION ( 'NONE',  ( 0.9609149988134837450, -0.1028163501681639419, 0.2570431154366518145 ) ) ;
#37006=DIRECTION ( 'NONE',  ( -0.000000000000000000, -0.9284778069183718952, -0.3713878862591649677 ) ) ;
#37007=EDGE_CURVE ( 'NONE', #4363, #32530, #16186, .T. ) ;
#37073=DIRECTION ( 'NONE',  ( -0.000000000000000000, -0.9284778069183718952, -0.3713878862591649677 ) ) ;
#37097=AXIS2_PLACEMENT_3D ( 'NONE', #18035, #28303, #38 ) ;
#37106=ORIENTED_EDGE ( 'NONE', *, *, #32785, .F. ) ;
#37114=CIRCLE ( 'NONE', #32749, 2.999999999999999556 ) ;
#37115=CARTESIAN_POINT ( 'NONE',  ( 67.30914723170953096, -51.38023326212514519, -34.64943124715581035 ) ) ;
#37126=ORIENTED_EDGE ( 'NONE', *, *, #238, .F. ) ;
#37137=EDGE_CURVE ( 'NONE', #36279, #34725, #44797, .T. ) ;
#37146=ORIENTED_EDGE ( 'NONE', *, *, #33755, .F. ) ;
#37165=EDGE_CURVE ( 'NONE', #13294, #14242, #10032, .T. ) ;
#37171=VERTEX_POINT ( 'NONE', #9340 ) ;
#37177=VECTOR ( 'NONE', #26673, 1000.000000000000000 ) ;
#37228=ORIENTED_EDGE ( 'NONE', *, *, #17337, .F. ) ;
#37234=ORIENTED_EDGE ( 'NONE', *, *, #21087, .T. ) ;
#37245=FACE_OUTER_BOUND ( 'NONE', #42217, .T. ) ;
#37250=DIRECTION ( 'NONE',  ( -0.000000000000000000, -0.9284778069183721172, -0.3713878862591650232 ) ) ;
#37257=CIRCLE ( 'NONE', #29983, 2.999999999999999556 ) ;
#37271=EDGE_CURVE ( 'NONE', #43627, #12584, #14105, .T. ) ;
#37272=DIRECTION ( 'NONE',  ( -0.2768435750659241079, -0.3568721902840695792, 0.8921882507333129819 ) ) ;
#37274=CONICAL_SURFACE ( 'NONE', #44597, 2.445500000000004448, 0.9599310885968757034 ) ;
#37294=ADVANCED_FACE ( 'NONE', ( #17524 ), #30952, .T. ) ;
#37301=VECTOR ( 'NONE', #8961, 1000.000000000000227 ) ;
#37304=DIRECTION ( 'NONE',  ( 0.9609149988134837450, -0.1028163501681639419, 0.2570431154366518145 ) ) ;
#37314=DIRECTION ( 'NONE',  ( -0.000000000000000000, -0.9284778069183721172, -0.3713878862591650232 ) ) ;
#37323=DIRECTION ( 'NONE',  ( 1.387778780781445676E-17, -0.9284778069183720062, -0.3713878862591650232 ) ) ;
#37344=CARTESIAN_POINT ( 'NONE',  ( 73.07463722459043254, -60.35343162539949446, -36.44966353086839206 ) ) ;
#37346=VECTOR ( 'NONE', #42764, 1000.000000000000114 ) ;
#37350=FILL_AREA_STYLE_COLOUR ( '', #18221 ) ;
#37354=EDGE_CURVE ( 'NONE', #12584, #39438, #44837, .T. ) ;
#37391=ORIENTED_EDGE ( 'NONE', *, *, #25429, .T. ) ;
#37400=CARTESIAN_POINT ( 'NONE',  ( 70.19189222814998175, -64.81574766768041229, -39.12908228425553858 ) ) ;
#37413=AXIS2_PLACEMENT_3D ( 'NONE', #29302, #15398, #19270 ) ;
#37423=VERTEX_POINT ( 'NONE', #35273 ) ;
#37434=DIRECTION ( 'NONE',  ( -0.000000000000000000, -0.9284778069183720062, -0.3713878862591650232 ) ) ;
#37456=VERTEX_POINT ( 'NONE', #14550 ) ;
#37466=ORIENTED_EDGE ( 'NONE', *, *, #8387, .T. ) ;
#37467=AXIS2_PLACEMENT_3D ( 'NONE', #35046, #31646, #3400 ) ;
#37490=DIRECTION ( 'NONE',  ( -0.000000000000000000, -0.9284778069183721172, -0.3713878862591650232 ) ) ;
#37495=CYLINDRICAL_SURFACE ( 'NONE', #34758, 3.000000000000001776 ) ;
#37499=EDGE_LOOP ( 'NONE', ( #2641, #13498, #4267, #4296, #13754 ) ) ;
#37507=CARTESIAN_POINT ( 'NONE',  ( 70.19189222814998175, -100.0979043305785581, -53.24182196210380624 ) ) ;
#37519=VERTEX_POINT ( 'NONE', #12489 ) ;
#37526=ORIENTED_EDGE ( 'NONE', *, *, #43751, .T. ) ;
#37538=DIRECTION ( 'NONE',  ( -0.000000000000000000, -0.9284778069183720062, -0.3713878862591650232 ) ) ;
#37539=CARTESIAN_POINT ( 'NONE',  ( 70.89841814381148311, -68.89136543047671069, -37.69090763720760151 ) ) ;
#37556=FACE_OUTER_BOUND ( 'NONE', #44484, .T. ) ;
#37559=EDGE_CURVE ( 'NONE', #33002, #16491, #29356, .T. ) ;
#37560=CIRCLE ( 'NONE', #23753, 2.999999999999999556 ) ;
#37576=EDGE_LOOP ( 'NONE', ( #44119, #21487, #11823, #9983, #37796 ) ) ;
#37577=CARTESIAN_POINT ( 'NONE',  ( 70.19189222814998175, -50.19222220871606766, -33.27972307567368659 ) ) ;
#37587=ADVANCED_FACE ( 'NONE', ( #4731 ), #8386, .T. ) ;
#37588=CIRCLE ( 'NONE', #12872, 2.999999999999999556 ) ;
#37596=DIRECTION ( 'NONE',  ( 0.9609149988134833009, -0.1028163501681649411, 0.2570431154366530913 ) ) ;
#37619=VECTOR ( 'NONE', #8168, 1000.000000000000227 ) ;
#37657=CARTESIAN_POINT ( 'NONE',  ( 70.89841814381148311, -71.67679885123182260, -38.80507129598510119 ) ) ;
#37676=AXIS2_PLACEMENT_3D ( 'NONE', #6980, #14715, #32254 ) ;
#37682=DIRECTION ( 'NONE',  ( -0.000000000000000000, -0.9284778069183718952, -0.3713878862591649677 ) ) ;
#37712=CARTESIAN_POINT ( 'NONE',  ( 71.02242295334774269, -52.47502135561418157, -37.29764242556413478 ) ) ;
#37714=ORIENTED_EDGE ( 'NONE', *, *, #29288, .T. ) ;
#37739=DIRECTION ( 'NONE',  ( -0.2768435750659241079, -0.3568721902840686355, 0.8921882507333134260 ) ) ;
#37774=CARTESIAN_POINT ( 'NONE',  ( 68.07789357685331311, -68.58957386525776201, -38.44539312525988350 ) ) ;
#37796=ORIENTED_EDGE ( 'NONE', *, *, #20558, .F. ) ;
#37798=ORIENTED_EDGE ( 'NONE', *, *, #41775, .T. ) ;
#37821=DIRECTION ( 'NONE',  ( 0.9609149988134837450, -0.1028163501681639419, 0.2570431154366518145 ) ) ;
#37837=CARTESIAN_POINT ( 'NONE',  ( 70.19189222814998175, -53.90613343638955968, -34.76527462071035046 ) ) ;
#37838=DIRECTION ( 'NONE',  ( 0.000000000000000000, 0.9284778069183720062, 0.3713878862591650232 ) ) ;
#37874=ORIENTED_EDGE ( 'NONE', *, *, #32414, .T. ) ;
#37878=DIRECTION ( 'NONE',  ( -0.9609149988134834119, 0.1028163501681648995, -0.2570431154366529802 ) ) ;
#37881=DIRECTION ( 'NONE',  ( 0.7871354856660198740, 0.4483307682966886643, 0.4235767337848242442 ) ) ;
#37911=AXIS2_PLACEMENT_3D ( 'NONE', #28383, #11058, #3974 ) ;
#37921=ORIENTED_EDGE ( 'NONE', *, *, #30678, .F. ) ;
#37963=DIRECTION ( 'NONE',  ( -0.000000000000000000, -0.9284778069183718952, -0.3713878862591649677 ) ) ;
#37976=ORIENTED_EDGE ( 'NONE', *, *, #6053, .F. ) ;
#37978=VECTOR ( 'NONE', #32172, 1000.000000000000000 ) ;
#37990=FACE_OUTER_BOUND ( 'NONE', #29312, .T. ) ;
#37996=DIRECTION ( 'NONE',  ( -0.2768435750659241079, -0.3568721902840695792, 0.8921882507333129819 ) ) ;
#38002=DIRECTION ( 'NONE',  ( -0.2768435750659253847, -0.3568721902840677473, 0.8921882507333133150 ) ) ;
#38023=DIRECTION ( 'NONE',  ( -0.000000000000000000, -0.9284778069183718952, -0.3713878862591649677 ) ) ;
#38026=EDGE_LOOP ( 'NONE', ( #24969, #44105, #5569, #22992, #37921 ) ) ;
#38041=LINE ( 'NONE', #406, #8191 ) ;
#38043=ORIENTED_EDGE ( 'NONE', *, *, #2447, .T. ) ;
#38052=AXIS2_PLACEMENT_3D ( 'NONE', #13577, #41177, #37272 ) ;
#38053=DIRECTION ( 'NONE',  ( -0.2768435750659239414, -0.3568721902840664151, 0.8921882507333142032 ) ) ;
#38059=EDGE_LOOP ( 'NONE', ( #23322, #20598, #18072, #15356, #29685 ) ) ;
#38065=PLANE ( 'NONE',  #10215 ) ;
#38074=ORIENTED_EDGE ( 'NONE', *, *, #34491, .T. ) ;
#38079=FACE_OUTER_BOUND ( 'NONE', #23137, .T. ) ;
#38081=DIRECTION ( 'NONE',  ( -0.2768435750659239414, -0.3568721902840664151, 0.8921882507333142032 ) ) ;
#38096=ORIENTED_EDGE ( 'NONE', *, *, #22804, .T. ) ;
#38098=VERTEX_POINT ( 'NONE', #10093 ) ;
#38114=CIRCLE ( 'NONE', #263, 2.541999999999999371 ) ;
#38120=ADVANCED_FACE ( 'NONE', ( #34232 ), #14255, .T. ) ;
#38125=EDGE_CURVE ( 'NONE', #5080, #34215, #29513, .T. ) ;
#38126=ADVANCED_FACE ( 'NONE', ( #30597 ), #252, .T. ) ;
#38158=EDGE_CURVE ( 'NONE', #41822, #29144, #27858, .T. ) ;
#38204=AXIS2_PLACEMENT_3D ( 'NONE', #35964, #31874, #14781 ) ;
#38211=DIRECTION ( 'NONE',  ( -0.000000000000000000, -0.9284778069183721172, -0.3713878862591650232 ) ) ;
#38216=DIRECTION ( 'NONE',  ( -0.000000000000000000, -0.9284778069183721172, -0.3713878862591650232 ) ) ;
#38222=LINE ( 'NONE', #30946, #36497 ) ;
#38240=VECTOR ( 'NONE', #29009, 1000.000000000000114 ) ;
#38263=CONICAL_SURFACE ( 'NONE', #34648, 2.999999999999999556, 0.9599310885968830309 ) ;
#38265=DIRECTION ( 'NONE',  ( -0.000000000000000000, -0.9284778069183721172, -0.3713878862591650232 ) ) ;
#38276=EDGE_CURVE ( 'NONE', #38683, #5080, #33, .T. ) ;
#38288=AXIS2_PLACEMENT_3D ( 'NONE', #39904, #8666, #29414 ) ;
#38296=DIRECTION ( 'NONE',  ( 0.000000000000000000, 0.9284778069183720062, 0.3713878862591650232 ) ) ;
#38303=ORIENTED_EDGE ( 'NONE', *, *, #23419, .T. ) ;
#38305=LINE ( 'NONE', #7690, #32547 ) ;
#38306=CARTESIAN_POINT ( 'NONE',  ( 67.30914723170953096, -60.66501133130886814, -38.36331010974746647 ) ) ;
#38310=ORIENTED_EDGE ( 'NONE', *, *, #38158, .F. ) ;
#38314=CARTESIAN_POINT ( 'NONE',  ( 70.19189222814998175, -55.19510675323109439, -35.28085945431567438 ) ) ;
#38317=CONICAL_SURFACE ( 'NONE', #15032, 2.445500000000004448, 0.9599310885968757034 ) ;
#38319=CARTESIAN_POINT ( 'NONE',  ( 70.19189222814998175, -100.0979043305785581, -53.24182196210380624 ) ) ;
#38344=VERTEX_POINT ( 'NONE', #38766 ) ;
#38361=CIRCLE ( 'NONE', #8536, 2.999999999999999556 ) ;
#38386=DIRECTION ( 'NONE',  ( 0.9609149988134843001, -0.1028163501681632064, 0.2570431154366505933 ) ) ;
#38401=CARTESIAN_POINT ( 'NONE',  ( 67.37136766119182596, -70.31694239570130378, -42.20474206142759499 ) ) ;
#38403=CARTESIAN_POINT ( 'NONE',  ( 70.19189222814998175, -100.0979043305785581, -53.24182196210380624 ) ) ;
#38424=LINE ( 'NONE', #27294, #1666 ) ;
#38450=LINE ( 'NONE', #3791, #5159 ) ;
#38453=CARTESIAN_POINT ( 'NONE',  ( 70.19189222814998175, -52.61716011954800365, -34.24968978710501943 ) ) ;
#38468=ORIENTED_EDGE ( 'NONE', *, *, #13318, .T. ) ;
#38525=VERTEX_POINT ( 'NONE', #4564 ) ;
#38534=LINE ( 'NONE', #7988, #26263 ) ;
#38540=CARTESIAN_POINT ( 'NONE',  ( 67.30914723170953096, -58.80805571747214344, -37.62053433722914519 ) ) ;
#38556=PLANE ( 'NONE',  #11925 ) ;
#38576=VECTOR ( 'NONE', #26837, 1000.000000000000000 ) ;
#38589=VECTOR ( 'NONE', #7722, 1000.000000000000000 ) ;
#38602=VECTOR ( 'NONE', #13944, 1000.000000000000227 ) ;
#38622=EDGE_CURVE ( 'NONE', #10810, #15070, #1156, .T. ) ;
#38630=EDGE_LOOP ( 'NONE', ( #32204, #20255, #16444, #7229 ) ) ;
#38637=CARTESIAN_POINT ( 'NONE',  ( 69.29215060918571112, -65.97558228610364495, -36.22947046937226645 ) ) ;
#38639=ADVANCED_FACE ( 'NONE', ( #18029 ), #41220, .T. ) ;
#38645=CARTESIAN_POINT ( 'NONE',  ( 70.19189222814998175, -62.62292920857806422, -38.25196254438899501 ) ) ;
#38646=DIRECTION ( 'NONE',  ( -0.000000000000000000, -0.9284778069183721172, -0.3713878862591650232 ) ) ;
#38658=LINE ( 'NONE', #4907, #45014 ) ;
#38663=ADVANCED_FACE ( 'NONE', ( #16191 ), #12831, .T. ) ;
#38681=EDGE_CURVE ( 'NONE', #2361, #42996, #1860, .T. ) ;
#38683=VERTEX_POINT ( 'NONE', #20516 ) ;
#38692=AXIS2_PLACEMENT_3D ( 'NONE', #14871, #28782, #15313 ) ;
#38701=AXIS2_PLACEMENT_3D ( 'NONE', #19395, #4806, #25350 ) ;
#38720=CARTESIAN_POINT ( 'NONE',  ( 70.19189222814998175, -54.47411573338475677, -34.99246555962335492 ) ) ;
#38724=EDGE_LOOP ( 'NONE', ( #19925, #39707, #9754, #44411, #10304 ) ) ;
#38729=ADVANCED_FACE ( 'NONE', ( #20957 ), #16513, .T. ) ;
#38744=CARTESIAN_POINT ( 'NONE',  ( 70.19189222814998175, -100.0979043305785581, -53.24182196210380624 ) ) ;
#38745=CARTESIAN_POINT ( 'NONE',  ( 68.42836698684014607, -67.15337231239986693, -42.03592829731906733 ) ) ;
#38753=CARTESIAN_POINT ( 'NONE',  ( 67.84197459855160162, -55.51165166589005651, -36.13664933202900897 ) ) ;
#38760=DIRECTION ( 'NONE',  ( -0.000000000000000000, -0.9284778069183718952, -0.3713878862591649677 ) ) ;
#38765=AXIS2_PLACEMENT_3D ( 'NONE', #11858, #910, #15496 ) ;
#38766=CARTESIAN_POINT ( 'NONE',  ( 69.51487126532624927, -51.06495315005575719, -31.09787670850536756 ) ) ;
#38774=ADVANCED_FACE ( 'NONE', ( #17100, #13226 ), #44917, .T. ) ;
#38796=AXIS2_PLACEMENT_3D ( 'NONE', #34307, #27034, #12910 ) ;
#38807=AXIS2_PLACEMENT_3D ( 'NONE', #31362, #23880, #6308 ) ;
#38877=DIRECTION ( 'NONE',  ( 0.9609149988134837450, -0.1028163501681639419, 0.2570431154366518145 ) ) ;
#38881=AXIS2_PLACEMENT_3D ( 'NONE', #40413, #27181, #2315 ) ;
#38882=DIRECTION ( 'NONE',  ( 0.9609149988134837450, -0.1028163501681639419, 0.2570431154366518145 ) ) ;
#38883=CARTESIAN_POINT ( 'NONE',  ( 73.07463722459043254, -53.85408697697087632, -33.84994832705423562 ) ) ;
#38889=ORIENTED_EDGE ( 'NONE', *, *, #27064, .T. ) ;
#38908=ORIENTED_EDGE ( 'NONE', *, *, #13061, .T. ) ;
#38918=ADVANCED_FACE ( 'NONE', ( #27799 ), #26898, .T. ) ;
#38922=ORIENTED_EDGE ( 'NONE', *, *, #25875, .F. ) ;
#38926=VERTEX_POINT ( 'NONE', #41051 ) ;
#38936=EDGE_CURVE ( 'NONE', #33632, #1444, #13453, .T. ) ;
#38952=DIRECTION ( 'NONE',  ( 0.9609149988134837450, -0.1028163501681639419, 0.2570431154366518145 ) ) ;
#38975=DIRECTION ( 'NONE',  ( -0.2768435750659243855, -0.3568721902840678029, 0.8921882507333135370 ) ) ;
#38993=EDGE_CURVE ( 'NONE', #26514, #35134, #37588, .T. ) ;
#39027=DIRECTION ( 'NONE',  ( 0.9609149988134837450, -0.1028163501681639419, 0.2570431154366518145 ) ) ;
#39037=CIRCLE ( 'NONE', #43409, 2.445500000000004448 ) ;
#39061=EDGE_CURVE ( 'NONE', #19163, #16083, #35966, .T. ) ;
#39066=CARTESIAN_POINT ( 'NONE',  ( 73.07463722459043254, -56.63952039772598823, -34.96411198583172819 ) ) ;
#39102=AXIS2_PLACEMENT_3D ( 'NONE', #27512, #42089, #27961 ) ;
#39112=DIRECTION ( 'NONE',  ( -0.000000000000000000, -0.9284778069183721172, -0.3713878862591650232 ) ) ;
#39117=DIRECTION ( 'NONE',  ( 0.9609149988134843001, -0.1028163501681632064, 0.2570431154366505933 ) ) ;
#39149=PRODUCT_CONTEXT ( 'NONE', #13723, 'mechanical' ) ;
#39161=DIRECTION ( 'NONE',  ( -0.2768435750659241079, -0.3568721902840695792, 0.8921882507333129819 ) ) ;
#39183=DIRECTION ( 'NONE',  ( -0.000000000000000000, -0.9284778069183718952, -0.3713878862591649677 ) ) ;
#39192=ORIENTED_EDGE ( 'NONE', *, *, #25875, .T. ) ;
#39223=ADVANCED_FACE ( 'NONE', ( #27752 ), #34564, .T. ) ;
#39241=ORIENTED_EDGE ( 'NONE', *, *, #2764, .T. ) ;
#39263=ADVANCED_FACE ( 'NONE', ( #13402 ), #38317, .T. ) ;
#39270=VECTOR ( 'NONE', #31993, 1000.000000000000227 ) ;
#39297=ORIENTED_EDGE ( 'NONE', *, *, #11637, .F. ) ;
#39307=ORIENTED_EDGE ( 'NONE', *, *, #3397, .T. ) ;
#39309=AXIS2_PLACEMENT_3D ( 'NONE', #42867, #14828, #42642 ) ;
#39337=AXIS2_PLACEMENT_3D ( 'NONE', #7014, #30734, #3367 ) ;
#39343=DIRECTION ( 'NONE',  ( -0.000000000000000000, -0.9284778069183721172, -0.3713878862591650232 ) ) ;
#39380=ADVANCED_FACE ( 'NONE', ( #30486 ), #44407, .T. ) ;
#39382=AXIS2_PLACEMENT_3D ( 'NONE', #28991, #42898, #11660 ) ;
#39392=ORIENTED_EDGE ( 'NONE', *, *, #4513, .F. ) ;
#39406=CIRCLE ( 'NONE', #11747, 2.999999999999999556 ) ;
#39419=ORIENTED_EDGE ( 'NONE', *, *, #29229, .F. ) ;
#39423=CARTESIAN_POINT ( 'NONE',  ( 67.84197459855160162, -59.22556289356354142, -37.62220087706567284 ) ) ;
#39430=EDGE_CURVE ( 'NONE', #38098, #15917, #18679, .T. ) ;
#39435=LINE ( 'NONE', #11177, #7005 ) ;
#39438=VERTEX_POINT ( 'NONE', #25219 ) ;
#39454=DIRECTION ( 'NONE',  ( 0.7871354856660198740, 0.4483307682966886643, 0.4235767337848242442 ) ) ;
#39481=EDGE_LOOP ( 'NONE', ( #28393, #10077 ) ) ;
#39511=CARTESIAN_POINT ( 'NONE',  ( 69.48815586033239811, -68.74046964786722924, -38.06815038123374251 ) ) ;
#39518=EDGE_CURVE ( 'NONE', #4027, #2361, #33201, .T. ) ;
#39519=ADVANCED_FACE ( 'NONE', ( #3775 ), #4460, .T. ) ;
#39523=CYLINDRICAL_SURFACE ( 'NONE', #27001, 3.000000000000001776 ) ;
#39524=AXIS2_PLACEMENT_3D ( 'NONE', #19913, #14126, #31666 ) ;
#39549=VERTEX_POINT ( 'NONE', #14953 ) ;
#39592=CARTESIAN_POINT ( 'NONE',  ( 71.02242295334774269, -99.02728775972636299, -55.91838671430374319 ) ) ;
#39604=AXIS2_PLACEMENT_3D ( 'NONE', #5840, #19764, #23417 ) ;
#39614=ORIENTED_EDGE ( 'NONE', *, *, #27807, .T. ) ;
#39627=CARTESIAN_POINT ( 'NONE',  ( 73.07463722459043254, -51.06865355621575731, -32.73578466827673594 ) ) ;
#39651=DIRECTION ( 'NONE',  ( -0.000000000000000000, -0.9284778069183718952, -0.3713878862591649677 ) ) ;
#39653=VERTEX_POINT ( 'NONE', #4001 ) ;
#39655=DIRECTION ( 'NONE',  ( -0.000000000000000000, -0.9284778069183721172, -0.3713878862591650232 ) ) ;
#39658=( NAMED_UNIT ( * ) PLANE_ANGLE_UNIT ( ) SI_UNIT ( $, .RADIAN. ) );
#39661=CARTESIAN_POINT ( 'NONE',  ( 70.19189222814998175, -70.34019061884472990, -41.33884020749756871 ) ) ;
#39707=ORIENTED_EDGE ( 'NONE', *, *, #41658, .F. ) ;
#39765=VERTEX_POINT ( 'NONE', #38883 ) ;
#39791=EDGE_CURVE ( 'NONE', #1762, #44794, #4171, .T. ) ;
#39823=FACE_OUTER_BOUND ( 'NONE', #5273, .T. ) ;
#39833=EDGE_CURVE ( 'NONE', #16121, #18545, #4677, .T. ) ;
#39837=DIRECTION ( 'NONE',  ( -0.000000000000000000, -0.9284778069183721172, -0.3713878862591650232 ) ) ;
#39839=ORIENTED_EDGE ( 'NONE', *, *, #25298, .T. ) ;
#39867=DIRECTION ( 'NONE',  ( 0.9609149988134837450, -0.1028163501681639419, 0.2570431154366518145 ) ) ;
#39890=VERTEX_POINT ( 'NONE', #42992 ) ;
#39904=CARTESIAN_POINT ( 'NONE',  ( 70.19189222814998175, -60.40547808481815650, -37.36498982452450690 ) ) ;
#39918=AXIS2_PLACEMENT_3D ( 'NONE', #25060, #14797, #4063 ) ;
#39956=ADVANCED_FACE ( 'NONE', ( #10149 ), #37495, .T. ) ;
#39970=ORIENTED_EDGE ( 'NONE', *, *, #26137, .T. ) ;
#40003=CARTESIAN_POINT ( 'NONE',  ( 67.30914723170953096, -54.16566668288025710, -35.76359490593331003 ) ) ;
#40022=ORIENTED_EDGE ( 'NONE', *, *, #38936, .F. ) ;
#40052=AXIS2_PLACEMENT_3D ( 'NONE', #38453, #4480, #10665 ) ;
#40055=FACE_OUTER_BOUND ( 'NONE', #40457, .T. ) ;
#40057=AXIS2_PLACEMENT_3D ( 'NONE', #40294, #36851, #5619 ) ;
#40106=CARTESIAN_POINT ( 'NONE',  ( 70.89841814381148311, -68.89136543047671069, -37.69090763720760151 ) ) ;
#40112=CARTESIAN_POINT ( 'NONE',  ( 70.19189222814998175, -67.83330054016514055, -40.33609291459782753 ) ) ;
#40137=ADVANCED_FACE ( 'NONE', ( #26289 ), #26781, .T. ) ;
#40157=ORIENTED_EDGE ( 'NONE', *, *, #7871, .F. ) ;
#40176=EDGE_LOOP ( 'NONE', ( #18015, #19931, #42426, #28286, #27755 ) ) ;
#40177=AXIS2_PLACEMENT_3D ( 'NONE', #28060, #31242, #454 ) ;
#40180=DIRECTION ( 'NONE',  ( 0.9609149988134837450, -0.1028163501681639419, 0.2570431154366518145 ) ) ;
#40181=EDGE_CURVE ( 'NONE', #9778, #2680, #20949, .T. ) ;
#40196=CARTESIAN_POINT ( 'NONE',  ( 69.36136150295220659, -54.61625449731858595, -31.94451292116425023 ) ) ;
#40200=ORIENTED_EDGE ( 'NONE', *, *, #28400, .F. ) ;
#40213=APPLICATION_CONTEXT ( 'automotive_design' ) ;
#40221=VERTEX_POINT ( 'NONE', #40196 ) ;
#40230=CARTESIAN_POINT ( 'NONE',  ( 72.54180985774836188, -55.08604862764417476, -34.50806356816917742 ) ) ;
#40235=DIRECTION ( 'NONE',  ( -0.7871354856660202071, 0.6167752151498580027, 0.002461946824133919541 ) ) ;
#40250=DIRECTION ( 'NONE',  ( -0.000000000000000000, -0.9284778069183721172, -0.3713878862591650232 ) ) ;
#40253=EDGE_CURVE ( 'NONE', #9298, #22284, #35854, .T. ) ;
#40287=CIRCLE ( 'NONE', #7527, 2.999999999999999556 ) ;
#40294=CARTESIAN_POINT ( 'NONE',  ( 70.19189222814998175, -61.90193818873174791, -37.96356864969668266 ) ) ;
#40298=DIRECTION ( 'NONE',  ( 0.9609149988134843001, -0.1028163501681632064, 0.2570431154366505933 ) ) ;
#40317=AXIS2_PLACEMENT_3D ( 'NONE', #23472, #43766, #9103 ) ;
#40329=VERTEX_POINT ( 'NONE', #8287 ) ;
#40333=PLANE ( 'NONE',  #909 ) ;
#40344=EDGE_CURVE ( 'NONE', #21214, #14508, #25313, .T. ) ;
#40352=CARTESIAN_POINT ( 'NONE',  ( 73.07463722459043254, -57.56799820464436834, -35.33549987209089238 ) ) ;
#40394=AXIS2_PLACEMENT_3D ( 'NONE', #30256, #40753, #23427 ) ;
#40399=EDGE_CURVE ( 'NONE', #27626, #22908, #302, .T. ) ;
#40413=CARTESIAN_POINT ( 'NONE',  ( 70.19189222814998175, -58.90901798090458641, -36.76641099935233825 ) ) ;
#40425=CARTESIAN_POINT ( 'NONE',  ( 70.19189222814998175, -70.61873396092025246, -41.45025657337532010 ) ) ;
#40431=EDGE_LOOP ( 'NONE', ( #5656, #26206, #22170, #20150, #3433 ) ) ;
#40457=EDGE_LOOP ( 'NONE', ( #28580, #3874, #15329, #2387, #1002, #22399 ) ) ;
#40458=FACE_OUTER_BOUND ( 'NONE', #40431, .T. ) ;
#40459=VECTOR ( 'NONE', #9007, 1000.000000000000114 ) ;
#40464=EDGE_CURVE ( 'NONE', #35202, #25805, #10137, .T. ) ;
#40466=AXIS2_PLACEMENT_3D ( 'NONE', #44398, #17464, #13162 ) ;
#40468=ORIENTED_EDGE ( 'NONE', *, *, #24542, .T. ) ;
#40505=ORIENTED_EDGE ( 'NONE', *, *, #15886, .F. ) ;
#40507=VECTOR ( 'NONE', #40812, 1000.000000000000227 ) ;
#40516=EDGE_CURVE ( 'NONE', #27773, #9431, #34714, .T. ) ;
#40529=CARTESIAN_POINT ( 'NONE',  ( 70.19189222814998175, -61.33395589173652951, -37.73637771078367109 ) ) ;
#40557=VERTEX_POINT ( 'NONE', #37712 ) ;
#40558=DIRECTION ( 'NONE',  ( -0.000000000000000000, -0.9284778069183721172, -0.3713878862591650232 ) ) ;
#40578=CIRCLE ( 'NONE', #39102, 2.445500000000001339 ) ;
#40618=CARTESIAN_POINT ( 'NONE',  ( 69.48536631248848039, -66.77523564985355620, -42.98127819198803934 ) ) ;
#40621=ORIENTED_EDGE ( 'NONE', *, *, #27064, .F. ) ;
#40635=CARTESIAN_POINT ( 'NONE',  ( 71.02242295334774269, -60.83132161787954573, -40.64013340189661960 ) ) ;
#40656=ORIENTED_EDGE ( 'NONE', *, *, #26390, .F. ) ;
#40670=CARTESIAN_POINT ( 'NONE',  ( 73.01241679510815175, -68.13509210538408922, -39.58160742654554554 ) ) ;
#40696=DIRECTION ( 'NONE',  ( 0.9609149988134837450, -0.1028163501681639419, 0.2570431154366518145 ) ) ;
#40718=FACE_OUTER_BOUND ( 'NONE', #44231, .T. ) ;
#40719=EDGE_CURVE ( 'NONE', #39549, #38098, #35502, .T. ) ;
#40747=VECTOR ( 'NONE', #13789, 1000.000000000000000 ) ;
#40753=DIRECTION ( 'NONE',  ( 0.000000000000000000, 0.9284778069183720062, 0.3713878862591650232 ) ) ;
#40755=EDGE_CURVE ( 'NONE', #38344, #43627, #38658, .T. ) ;
#40792=SURFACE_SIDE_STYLE ('',( #26876 ) ) ;
#40794=DIRECTION ( 'NONE',  ( -0.2768435750659241079, -0.3568721902840686355, 0.8921882507333134260 ) ) ;
#40809=DIRECTION ( 'NONE',  ( -0.2768435750659241079, -0.3568721902840695792, 0.8921882507333129819 ) ) ;
#40812=DIRECTION ( 'NONE',  ( -0.000000000000000000, -0.9284778069183718952, -0.3713878862591649677 ) ) ;
#40818=CARTESIAN_POINT ( 'NONE',  ( 70.19189222814998175, -100.0979043305785581, -53.24182196210380624 ) ) ;
#40842=CARTESIAN_POINT ( 'NONE',  ( 71.02242295334774269, -55.98144579621563821, -38.70019997903393971 ) ) ;
#40859=CIRCLE ( 'NONE', #2226, 2.445500000000004448 ) ;
#40898=CYLINDRICAL_SURFACE ( 'NONE', #11699, 3.000000000000001776 ) ;
#40910=ORIENTED_EDGE ( 'NONE', *, *, #26803, .T. ) ;
#40911=EDGE_CURVE ( 'NONE', #30461, #11921, #31158, .T. ) ;
#40938=DIRECTION ( 'NONE',  ( -0.000000000000000000, -0.9284778069183718952, -0.3713878862591649677 ) ) ;
#40991=CARTESIAN_POINT ( 'NONE',  ( 70.19189222814998175, -52.04917782255280656, -34.02249884819201498 ) ) ;
#41015=ORIENTED_EDGE ( 'NONE', *, *, #27018, .T. ) ;
#41021=ORIENTED_EDGE ( 'NONE', *, *, #12796, .F. ) ;
#41048=DIRECTION ( 'NONE',  ( 0.9609149988134837450, -0.1028163501681639419, 0.2570431154366518145 ) ) ;
#41051=CARTESIAN_POINT ( 'NONE',  ( 69.36136150295220659, -65.88636423853262158, -36.45251753205559453 ) ) ;
#41066=ORIENTED_EDGE ( 'NONE', *, *, #7862, .F. ) ;
#41097=VERTEX_POINT ( 'NONE', #5807 ) ;
#41101=DIRECTION ( 'NONE',  ( 0.9609149988134837450, -0.1028163501681639419, 0.2570431154366518145 ) ) ;
#41102=DIRECTION ( 'NONE',  ( -0.000000000000000000, -0.9284778069183721172, -0.3713878862591650232 ) ) ;
#41130=AXIS2_PLACEMENT_3D ( 'NONE', #29688, #43600, #40180 ) ;
#41154=DIRECTION ( 'NONE',  ( -0.000000000000000000, -0.9284778069183720062, -0.3713878862591650232 ) ) ;
#41177=DIRECTION ( 'NONE',  ( -0.000000000000000000, -0.9284778069183718952, -0.3713878862591649677 ) ) ;
#41180=CARTESIAN_POINT ( 'NONE',  ( 67.30914723170953096, -56.02262229671700311, -36.50637067845163841 ) ) ;
#41211=( NAMED_UNIT ( * ) SI_UNIT ( $, .STERADIAN. ) SOLID_ANGLE_UNIT ( ) );
#41220=CONICAL_SURFACE ( 'NONE', #12108, 2.445500000000004448, 0.9599310885968757034 ) ;
#41224=ORIENTED_EDGE ( 'NONE', *, *, #32785, .T. ) ;
#41246=ADVANCED_FACE ( 'NONE', ( #40718 ), #13132, .T. ) ;
#41248=ORIENTED_EDGE ( 'NONE', *, *, #12380, .F. ) ;
#41255=SURFACE_STYLE_USAGE ( .BOTH. , #40792 ) ;
#41256=CARTESIAN_POINT ( 'NONE',  ( 70.19189222814998175, -65.04786711941001442, -39.22192925582032785 ) ) ;
#41276=CARTESIAN_POINT ( 'NONE',  ( 70.19189222814998175, -60.97346038181336070, -37.59218076343751136 ) ) ;
#41286=EDGE_CURVE ( 'NONE', #9213, #31092, #25892, .T. ) ;
#41338=DIRECTION ( 'NONE',  ( 0.9609149988134843001, -0.1028163501681632064, 0.2570431154366505933 ) ) ;
#41357=DIRECTION ( 'NONE',  ( -0.000000000000000000, -0.9284778069183721172, -0.3713878862591650232 ) ) ;
#41382=DIRECTION ( 'NONE',  ( -0.000000000000000000, -0.9284778069183718952, -0.3713878862591649677 ) ) ;
#41392=ORIENTED_EDGE ( 'NONE', *, *, #25873, .T. ) ;
#41411=EDGE_CURVE ( 'NONE', #4363, #27773, #25187, .T. ) ;
#41413=AXIS2_PLACEMENT_3D ( 'NONE', #24830, #21409, #17764 ) ;
#41426=ORIENTED_EDGE ( 'NONE', *, *, #3028, .F. ) ;
#41440=CARTESIAN_POINT ( 'NONE',  ( 69.29215060918571112, -66.20770173783323287, -36.32231744093705572 ) ) ;
#41457=CARTESIAN_POINT ( 'NONE',  ( 70.89841814381148311, -68.89136543047671069, -37.69090763720760151 ) ) ;
#41493=EDGE_CURVE ( 'NONE', #33632, #25485, #24465, .T. ) ;
#41495=DIRECTION ( 'NONE',  ( -0.000000000000000000, -0.9284778069183721172, -0.3713878862591650232 ) ) ;
#41514=DIRECTION ( 'NONE',  ( 0.9609149988134843001, -0.1028163501681632064, 0.2570431154366505933 ) ) ;
#41534=ORIENTED_EDGE ( 'NONE', *, *, #41286, .F. ) ;
#41540=ORIENTED_EDGE ( 'NONE', *, *, #6611, .T. ) ;
#41544=LINE ( 'NONE', #37657, #4446 ) ;
#41555=ADVANCED_FACE ( 'NONE', ( #24510 ), #26675, .T. ) ;
#41560=DIRECTION ( 'NONE',  ( -0.2768435750659263839, -0.3568721902840679139, 0.8921882507333128709 ) ) ;
#41567=ORIENTED_EDGE ( 'NONE', *, *, #40719, .F. ) ;
#41576=EDGE_LOOP ( 'NONE', ( #628, #10519, #37391, #13462, #34327 ) ) ;
#41577=DIRECTION ( 'NONE',  ( -0.000000000000000000, -0.9284778069183721172, -0.3713878862591650232 ) ) ;
#41583=VECTOR ( 'NONE', #5591, 1000.000000000000227 ) ;
#41585=UNCERTAINTY_MEASURE_WITH_UNIT (LENGTH_MEASURE( 1.000000000000000082E-05 ), #23464, 'distance_accuracy_value', 'NONE');
#41591=DIRECTION ( 'NONE',  ( -0.2407039305251456596, 0.3604685577742790525, -0.9011792478113757054 ) ) ;
#41594=CARTESIAN_POINT ( 'NONE',  ( 70.19189222814998175, -58.18802696105826300, -36.47801710466001879 ) ) ;
#41601=ORIENTED_EDGE ( 'NONE', *, *, #43691, .F. ) ;
#41607=EDGE_CURVE ( 'NONE', #9213, #44499, #769, .T. ) ;
#41608=CYLINDRICAL_SURFACE ( 'NONE', #43796, 5.000000000000002665 ) ;
#41658=EDGE_CURVE ( 'NONE', #8943, #20803, #39037, .T. ) ;
#41662=CARTESIAN_POINT ( 'NONE',  ( 70.19189222814998175, -50.76020450571126474, -33.50691401458669105 ) ) ;
#41673=DIRECTION ( 'NONE',  ( -0.2768435750659253847, -0.3568721902840677473, 0.8921882507333133150 ) ) ;
#41702=ORIENTED_EDGE ( 'NONE', *, *, #25429, .F. ) ;
#41723=CIRCLE ( 'NONE', #19153, 0.2499999999999990841 ) ;
#41730=LINE ( 'NONE', #17771, #193 ) ;
#41758=ORIENTED_EDGE ( 'NONE', *, *, #33350, .T. ) ;
#41775=EDGE_CURVE ( 'NONE', #44431, #18777, #17915, .T. ) ;
#41776=ORIENTED_EDGE ( 'NONE', *, *, #8870, .T. ) ;
#41777=AXIS2_PLACEMENT_3D ( 'NONE', #39661, #42414, #38975 ) ;
#41779=DIRECTION ( 'NONE',  ( 0.9609149988134839671, -0.1028163501681660097, 0.2570431154366504822 ) ) ;
#41792=FACE_OUTER_BOUND ( 'NONE', #33407, .T. ) ;
#41798=CIRCLE ( 'NONE', #39604, 2.999999999999999556 ) ;
#41822=VERTEX_POINT ( 'NONE', #26531 ) ;
#41829=DIRECTION ( 'NONE',  ( 0.000000000000000000, 0.9284778069183720062, 0.3713878862591650232 ) ) ;
#41845=DIRECTION ( 'NONE',  ( 0.9609149988134833009, -0.1028163501681649411, 0.2570431154366530913 ) ) ;
#41863=ORIENTED_EDGE ( 'NONE', *, *, #30988, .F. ) ;
#41866=AXIS2_PLACEMENT_3D ( 'NONE', #27529, #24549, #42327 ) ;
#41875=CYLINDRICAL_SURFACE ( 'NONE', #314, 3.000000000000001776 ) ;
#41921=AXIS2_PLACEMENT_3D ( 'NONE', #38319, #3006, #44514 ) ;
#41926=FACE_OUTER_BOUND ( 'NONE', #27329, .T. ) ;
#41964=FACE_OUTER_BOUND ( 'NONE', #27238, .T. ) ;
#41995=ORIENTED_EDGE ( 'NONE', *, *, #3802, .F. ) ;
#42003=EDGE_LOOP ( 'NONE', ( #41601, #19302, #38074, #34334, #11009 ) ) ;
#42022=ORIENTED_EDGE ( 'NONE', *, *, #33091, .T. ) ;
#42038=FACE_OUTER_BOUND ( 'NONE', #37576, .T. ) ;
#42040=ORIENTED_EDGE ( 'NONE', *, *, #39061, .F. ) ;
#42089=DIRECTION ( 'NONE',  ( -0.000000000000000000, -0.9284778069183721172, -0.3713878862591650232 ) ) ;
#42098=EDGE_CURVE ( 'NONE', #19823, #33002, #14311, .T. ) ;
#42106=AXIS2_PLACEMENT_3D ( 'NONE', #23267, #45145, #27368 ) ;
#42139=AXIS2_PLACEMENT_3D ( 'NONE', #37577, #2917, #16618 ) ;
#42147=EDGE_LOOP ( 'NONE', ( #22046, #4327, #19402, #11315, #2456 ) ) ;
#42167=DIRECTION ( 'NONE',  ( -0.000000000000000000, -0.9284778069183721172, -0.3713878862591650232 ) ) ;
#42169=CARTESIAN_POINT ( 'NONE',  ( 70.19189222814998175, -57.98054017398621340, -36.39502311309316696 ) ) ;
#42185=CARTESIAN_POINT ( 'NONE',  ( 0.000000000000000000, 0.000000000000000000, 0.000000000000000000 ) ) ;
#42187=DIRECTION ( 'NONE',  ( -0.2768435750659241079, -0.3568721902840695792, 0.8921882507333129819 ) ) ;
#42192=CARTESIAN_POINT ( 'NONE',  ( 70.19189222814998175, -52.40967333247598248, -34.16669579553818181 ) ) ;
#42195=ORIENTED_EDGE ( 'NONE', *, *, #28095, .F. ) ;
#42204=CIRCLE ( 'NONE', #13089, 2.999999999999999556 ) ;
#42210=DIRECTION ( 'NONE',  ( 0.9609149988134837450, -0.1028163501681639419, 0.2570431154366518145 ) ) ;
#42217=EDGE_LOOP ( 'NONE', ( #33524, #40468, #14792, #35066, #2812 ) ) ;
#42219=DIRECTION ( 'NONE',  ( -0.000000000000000000, -0.9284778069183718952, -0.3713878862591649677 ) ) ;
#42239=CIRCLE ( 'NONE', #32026, 2.999999999999999556 ) ;
#42249=ORIENTED_EDGE ( 'NONE', *, *, #238, .T. ) ;
#42258=DIRECTION ( 'NONE',  ( 0.9609149988134843001, -0.1028163501681632064, 0.2570431154366505933 ) ) ;
#42261=CARTESIAN_POINT ( 'NONE',  ( 72.54180985774836188, -57.87148204839928667, -35.62222722694667709 ) ) ;
#42271=CARTESIAN_POINT ( 'NONE',  ( 70.19189222814998175, -100.0979043305785581, -53.24182196210380624 ) ) ;
#42276=ORIENTED_EDGE ( 'NONE', *, *, #43882, .T. ) ;
#42285=DIRECTION ( 'NONE',  ( -0.000000000000000000, -0.9284778069183721172, -0.3713878862591650232 ) ) ;
#42319=CARTESIAN_POINT ( 'NONE',  ( 70.19189222814998175, -58.54852247098141049, -36.62221405200617141 ) ) ;
#42324=EDGE_CURVE ( 'NONE', #18078, #32530, #24498, .T. ) ;
#42327=DIRECTION ( 'NONE',  ( 0.9609149988134837450, -0.1028163501681639419, 0.2570431154366518145 ) ) ;
#42353=DIRECTION ( 'NONE',  ( 0.9609149988134837450, -0.1028163501681639419, 0.2570431154366518145 ) ) ;
#42365=CARTESIAN_POINT ( 'NONE',  ( 70.19189222814998175, -57.98054017398621340, -36.39502311309316696 ) ) ;
#42384=CARTESIAN_POINT ( 'NONE',  ( 70.19189222814998175, -60.97346038181336070, -37.59218076343751136 ) ) ;
#42404=CIRCLE ( 'NONE', #22728, 2.999999999999999556 ) ;
#42412=CARTESIAN_POINT ( 'NONE',  ( 73.07463722459043254, -62.00290045216418378, -37.10944531181986861 ) ) ;
#42414=DIRECTION ( 'NONE',  ( -0.000000000000000000, -0.9284778069183718952, -0.3713878862591649677 ) ) ;
#42426=ORIENTED_EDGE ( 'NONE', *, *, #18739, .F. ) ;
#42441=VERTEX_POINT ( 'NONE', #21707 ) ;
#42457=AXIS2_PLACEMENT_3D ( 'NONE', #1610, #19624, #19180 ) ;
#42481=VERTEX_POINT ( 'NONE', #25578 ) ;
#42488=VECTOR ( 'NONE', #13250, 1000.000000000000000 ) ;
#42493=EDGE_CURVE ( 'NONE', #43396, #29748, #44204, .T. ) ;
#42497=DIRECTION ( 'NONE',  ( 0.9609149988134837450, -0.1028163501681639419, 0.2570431154366518145 ) ) ;
#42543=DIRECTION ( 'NONE',  ( 0.9609149988134837450, -0.1028163501681639419, 0.2570431154366518145 ) ) ;
#42611=AXIS2_PLACEMENT_3D ( 'NONE', #25442, #38646, #28637 ) ;
#42616=DIRECTION ( 'NONE',  ( -0.000000000000000000, -0.9284778069183721172, -0.3713878862591650232 ) ) ;
#42620=ORIENTED_EDGE ( 'NONE', *, *, #37165, .F. ) ;
#42642=DIRECTION ( 'NONE',  ( 0.9609149988134837450, -0.1028163501681639419, 0.2570431154366518145 ) ) ;
#42672=VERTEX_POINT ( 'NONE', #8691 ) ;
#42679=CARTESIAN_POINT ( 'NONE',  ( 70.19189222814998175, -70.61873396092025246, -41.45025657337532010 ) ) ;
#42680=AXIS2_PLACEMENT_3D ( 'NONE', #1693, #29740, #32698 ) ;
#42696=CARTESIAN_POINT ( 'NONE',  ( 67.30914723170953096, -61.59348913822725535, -38.73469799600663777 ) ) ;
#42729=ORIENTED_EDGE ( 'NONE', *, *, #22838, .T. ) ;
#42740=CARTESIAN_POINT ( 'NONE',  ( 70.19189222814998175, -59.47700027789979060, -36.99360193826534271 ) ) ;
#42764=DIRECTION ( 'NONE',  ( -0.7871354856660202071, 0.6167752151498580027, 0.002461946824133919541 ) ) ;
#42766=CONICAL_SURFACE ( 'NONE', #27475, 2.445500000000004448, 0.9599310885968757034 ) ;
#42803=CARTESIAN_POINT ( 'NONE',  ( 70.19189222814998175, -51.68868231262963775, -33.87830190084585524 ) ) ;
#42814=DIRECTION ( 'NONE',  ( -0.000000000000000000, -0.9284778069183721172, -0.3713878862591650232 ) ) ;
#42819=CARTESIAN_POINT ( 'NONE',  ( 71.02242295334774269, -55.05296798929726521, -38.32881209277477552 ) ) ;
#42822=CARTESIAN_POINT ( 'NONE',  ( 70.19189222814998175, -55.19510675323109439, -35.28085945431567438 ) ) ;
#42845=EDGE_LOOP ( 'NONE', ( #41021, #22315, #3589, #25797, #29604 ) ) ;
#42857=DIRECTION ( 'NONE',  ( -0.000000000000000000, -0.9284778069183718952, -0.3713878862591649677 ) ) ;
#42858=CYLINDRICAL_SURFACE ( 'NONE', #9222, 3.000000000000001776 ) ;
#42867=CARTESIAN_POINT ( 'NONE',  ( 70.19189222814998175, -61.69445140165969121, -37.88057465812982372 ) ) ;
#42898=DIRECTION ( 'NONE',  ( -0.000000000000000000, -0.9284778069183721172, -0.3713878862591650232 ) ) ;
#42902=DIRECTION ( 'NONE',  ( 1.387778780781445676E-17, -0.9284778069183720062, -0.3713878862591650232 ) ) ;
#42921=AXIS2_PLACEMENT_3D ( 'NONE', #1437, #25626, #8516 ) ;
#42947=ORIENTED_EDGE ( 'NONE', *, *, #34508, .F. ) ;
#42961=AXIS2_PLACEMENT_3D ( 'NONE', #29254, #4403, #35628 ) ;
#42967=ORIENTED_EDGE ( 'NONE', *, *, #3275, .T. ) ;
#42981=CIRCLE ( 'NONE', #17502, 2.999999999999999556 ) ;
#42992=CARTESIAN_POINT ( 'NONE',  ( 71.02242295334774269, -51.33905676162378739, -36.84326054773811876 ) ) ;
#42996=VERTEX_POINT ( 'NONE', #13098 ) ;
#43007=CARTESIAN_POINT ( 'NONE',  ( 67.84197459855160162, -62.01099631431865333, -38.73636453584316541 ) ) ;
#43009=DIRECTION ( 'NONE',  ( -0.000000000000000000, -0.9284778069183718952, -0.3713878862591649677 ) ) ;
#43012=DIRECTION ( 'NONE',  ( 0.7202110682883375858, 0.2576522076061144029, -0.6441361323747234469 ) ) ;
#43018=CARTESIAN_POINT ( 'NONE',  ( 67.30914723170953096, -51.38023326212514519, -34.64943124715581035 ) ) ;
#43051=VECTOR ( 'NONE', #22324, 1000.000000000000227 ) ;
#43081=ORIENTED_EDGE ( 'NONE', *, *, #29924, .T. ) ;
#43092=ORIENTED_EDGE ( 'NONE', *, *, #9672, .T. ) ;
#43126=ORIENTED_EDGE ( 'NONE', *, *, #29888, .F. ) ;
#43147=AXIS2_PLACEMENT_3D ( 'NONE', #4287, #1098, #11595 ) ;
#43152=ADVANCED_FACE ( 'NONE', ( #9438 ), #26997, .T. ) ;
#43169=AXIS2_PLACEMENT_3D ( 'NONE', #5140, #19056, #32942 ) ;
#43177=DIRECTION ( 'NONE',  ( -0.000000000000000000, -0.9284778069183721172, -0.3713878862591650232 ) ) ;
#43180=ADVANCED_FACE ( 'NONE', ( #40458 ), #18701, .T. ) ;
#43188=CARTESIAN_POINT ( 'NONE',  ( 73.07463722459043254, -62.21038723923624048, -37.19243930338672754 ) ) ;
#43201=ORIENTED_EDGE ( 'NONE', *, *, #24599, .F. ) ;
#43203=AXIS2_PLACEMENT_3D ( 'NONE', #19357, #22327, #19580 ) ;
#43210=CIRCLE ( 'NONE', #3879, 2.541999999999999371 ) ;
#43260=DIRECTION ( 'NONE',  ( -0.000000000000000000, -0.9284778069183718952, -0.3713878862591649677 ) ) ;
#43266=ORIENTED_EDGE ( 'NONE', *, *, #1925, .T. ) ;
#43271=CARTESIAN_POINT ( 'NONE',  ( 72.54180985774836188, -60.65691546915440568, -36.73639088572416966 ) ) ;
#43312=ORIENTED_EDGE ( 'NONE', *, *, #26228, .F. ) ;
#43315=LINE ( 'NONE', #25091, #44629 ) ;
#43320=CARTESIAN_POINT ( 'NONE',  ( 70.19189222814998175, -59.11650476797663600, -36.84940499091918298 ) ) ;
#43352=AXIS2_PLACEMENT_3D ( 'NONE', #31482, #14161, #33369 ) ;
#43362=VECTOR ( 'NONE', #6184, 999.9999999999998863 ) ;
#43396=VERTEX_POINT ( 'NONE', #27681 ) ;
#43409=AXIS2_PLACEMENT_3D ( 'NONE', #42740, #4194, #25409 ) ;
#43415=ADVANCED_FACE ( 'NONE', ( #7135 ), #2678, .T. ) ;
#43419=EDGE_CURVE ( 'NONE', #12164, #26262, #26714, .T. ) ;
#43429=LINE ( 'NONE', #40230, #1250 ) ;
#43443=ORIENTED_EDGE ( 'NONE', *, *, #3802, .T. ) ;
#43487=CARTESIAN_POINT ( 'NONE',  ( 70.19189222814998175, -54.26662894631272849, -34.90947156805651019 ) ) ;
#43489=VERTEX_POINT ( 'NONE', #43591 ) ;
#43493=CARTESIAN_POINT ( 'NONE',  ( 70.19189222814998175, -100.0979043305785581, -53.24182196210380624 ) ) ;
#43508=ORIENTED_EDGE ( 'NONE', *, *, #44296, .F. ) ;
#43518=DIRECTION ( 'NONE',  ( -0.7871354856660202071, 0.6167752151498580027, 0.002461946824133919541 ) ) ;
#43523=AXIS2_PLACEMENT_3D ( 'NONE', #30885, #16309, #5798 ) ;
#43561=ORIENTED_EDGE ( 'NONE', *, *, #5394, .T. ) ;
#43591=CARTESIAN_POINT ( 'NONE',  ( 73.07463722459043254, -58.49647601156275556, -35.70688775835006368 ) ) ;
#43600=DIRECTION ( 'NONE',  ( -0.000000000000000000, -0.9284778069183721172, -0.3713878862591650232 ) ) ;
#43603=DIRECTION ( 'NONE',  ( -0.2397535688815953248, -0.7732992861493835912, 0.5869637469634660931 ) ) ;
#43616=DIRECTION ( 'NONE',  ( -0.2768435750659266059, -0.3568721902840680249, 0.8921882507333128709 ) ) ;
#43627=VERTEX_POINT ( 'NONE', #25147 ) ;
#43634=AXIS2_PLACEMENT_3D ( 'NONE', #21972, #23101, #16722 ) ;
#43639=ORIENTED_EDGE ( 'NONE', *, *, #9118, .F. ) ;
#43653=AXIS2_PLACEMENT_3D ( 'NONE', #44072, #37434, #12836 ) ;
#43691=EDGE_CURVE ( 'NONE', #10336, #3754, #38305, .T. ) ;
#43692=DIRECTION ( 'NONE',  ( 0.7871354856660198740, 0.4483307682966886643, 0.4235767337848242442 ) ) ;
#43697=AXIS2_PLACEMENT_3D ( 'NONE', #23956, #37838, #6615 ) ;
#43710=ORIENTED_EDGE ( 'NONE', *, *, #16992, .F. ) ;
#43711=CIRCLE ( 'NONE', #24064, 2.445500000000004448 ) ;
#43724=CARTESIAN_POINT ( 'NONE',  ( 70.19189222814998175, -54.83461124330791847, -35.13666250696951465 ) ) ;
#43726=ADVANCED_FACE ( 'NONE', ( #8374 ), #5165, .T. ) ;
#43751=EDGE_CURVE ( 'NONE', #35294, #13294, #9272, .T. ) ;
#43754=CARTESIAN_POINT ( 'NONE',  ( 70.19189222814998175, -100.0979043305785581, -53.24182196210380624 ) ) ;
#43766=DIRECTION ( 'NONE',  ( 0.000000000000000000, 0.9284778069183720062, 0.3713878862591650232 ) ) ;
#43773=CONICAL_SURFACE ( 'NONE', #11744, 2.999999999999999556, 0.9599310885968830309 ) ;
#43776=CARTESIAN_POINT ( 'NONE',  ( 67.30914723170953096, -56.95110010363538322, -36.87775856471080260 ) ) ;
#43777=AXIS2_PLACEMENT_3D ( 'NONE', #7753, #22114, #7523 ) ;
#43796=AXIS2_PLACEMENT_3D ( 'NONE', #20842, #16987, #6935 ) ;
#43816=ADVANCED_FACE ( 'NONE', ( #3329 ), #13636, .F. ) ;
#43830=ORIENTED_EDGE ( 'NONE', *, *, #7604, .F. ) ;
#43863=CIRCLE ( 'NONE', #17650, 4.699999999999999289 ) ;
#43882=EDGE_CURVE ( 'NONE', #41097, #12584, #34720, .T. ) ;
#43937=VECTOR ( 'NONE', #12307, 1000.000000000000227 ) ;
#43941=EDGE_LOOP ( 'NONE', ( #18879, #29509, #30636, #19191, #31101, #17704 ) ) ;
#43944=LINE ( 'NONE', #12709, #31300 ) ;
#43967=CIRCLE ( 'NONE', #989, 2.999999999999999556 ) ;
#43981=ORIENTED_EDGE ( 'NONE', *, *, #45138, .F. ) ;
#43985=DIRECTION ( 'NONE',  ( 0.000000000000000000, 0.9284778069183720062, 0.3713878862591650232 ) ) ;
#43991=EDGE_CURVE ( 'NONE', #38344, #9298, #40578, .T. ) ;
#43994=ORIENTED_EDGE ( 'NONE', *, *, #20658, .F. ) ;
#44005=DIRECTION ( 'NONE',  ( 0.7871354856660198740, 0.4483307682966886643, 0.4235767337848242442 ) ) ;
#44006=EDGE_CURVE ( 'NONE', #19823, #4387, #35671, .T. ) ;
#44007=EDGE_CURVE ( 'NONE', #32876, #4821, #21622, .T. ) ;
#44035=DIRECTION ( 'NONE',  ( 0.9609149988134837450, -0.1028163501681639419, 0.2570431154366518145 ) ) ;
#44070=EDGE_CURVE ( 'NONE', #13382, #11921, #43429, .T. ) ;
#44072=CARTESIAN_POINT ( 'NONE',  ( 70.19189222814998175, -52.97765562947117957, -34.39388673445118627 ) ) ;
#44086=CYLINDRICAL_SURFACE ( 'NONE', #35040, 3.000000000000001776 ) ;
#44094=ORIENTED_EDGE ( 'NONE', *, *, #30928, .T. ) ;
#44105=ORIENTED_EDGE ( 'NONE', *, *, #9520, .T. ) ;
#44119=ORIENTED_EDGE ( 'NONE', *, *, #4967, .F. ) ;
#44160=CIRCLE ( 'NONE', #11405, 2.999999999999999556 ) ;
#44165=EDGE_LOOP ( 'NONE', ( #15898, #41534, #35939, #12053, #9162 ) ) ;
#44173=DIRECTION ( 'NONE',  ( -0.2768435750659241079, -0.3568721902840695792, 0.8921882507333129819 ) ) ;
#44177=AXIS2_PLACEMENT_3D ( 'NONE', #24332, #38216, #27976 ) ;
#44186=LINE ( 'NONE', #27526, #33272 ) ;
#44203=CARTESIAN_POINT ( 'NONE',  ( 73.07463722459043254, -55.50355580373558695, -34.50973010800571927 ) ) ;
#44204=CIRCLE ( 'NONE', #1216, 2.999999999999999556 ) ;
#44211=ORIENTED_EDGE ( 'NONE', *, *, #30653, .T. ) ;
#44214=CIRCLE ( 'NONE', #1227, 2.999999999999999556 ) ;
#44231=EDGE_LOOP ( 'NONE', ( #2872, #21161, #26085, #21255, #26759, #14169 ) ) ;
#44236=DIRECTION ( 'NONE',  ( 0.9609149988134837450, -0.1028163501681639419, 0.2570431154366518145 ) ) ;
#44290=ORIENTED_EDGE ( 'NONE', *, *, #13048, .F. ) ;
#44294=CARTESIAN_POINT ( 'NONE',  ( 70.19189222814998175, -53.54563792646638376, -34.62107767336419073 ) ) ;
#44296=EDGE_CURVE ( 'NONE', #36562, #40329, #28216, .T. ) ;
#44303=ORIENTED_EDGE ( 'NONE', *, *, #12554, .T. ) ;
#44346=DIRECTION ( 'NONE',  ( -0.000000000000000000, -0.9284778069183721172, -0.3713878862591650232 ) ) ;
#44348=CARTESIAN_POINT ( 'NONE',  ( 70.19189222814998175, -60.97346038181336070, -37.59218076343751136 ) ) ;
#44353=CARTESIAN_POINT ( 'NONE',  ( 67.84197459855160162, -58.29708508664516842, -37.25081299080650865 ) ) ;
#44398=CARTESIAN_POINT ( 'NONE',  ( 70.19189222814998175, -59.47700027789979060, -36.99360193826534271 ) ) ;
#44407=CYLINDRICAL_SURFACE ( 'NONE', #30328, 3.000000000000001776 ) ;
#44411=ORIENTED_EDGE ( 'NONE', *, *, #10836, .T. ) ;
#44425=ORIENTED_EDGE ( 'NONE', *, *, #23925, .F. ) ;
#44431=VERTEX_POINT ( 'NONE', #1750 ) ;
#44432=CARTESIAN_POINT ( 'NONE',  ( 70.86891319097370001, -49.31949126737637812, -35.46156944284200563 ) ) ;
#44440=CONICAL_SURFACE ( 'NONE', #40057, 2.999999999999999556, 0.9599310885968830309 ) ;
#44441=CARTESIAN_POINT ( 'NONE',  ( 71.02242295334774269, -56.90992360313401122, -39.07158786529310390 ) ) ;
#44451=VERTEX_POINT ( 'NONE', #36627 ) ;
#44456=CARTESIAN_POINT ( 'NONE',  ( 70.19189222814998175, -61.90193818873174791, -37.96356864969668266 ) ) ;
#44460=DIRECTION ( 'NONE',  ( -0.000000000000000000, -0.9284778069183718952, -0.3713878862591649677 ) ) ;
#44462=AXIS2_PLACEMENT_3D ( 'NONE', #27856, #17587, #251 ) ;
#44476=ORIENTED_EDGE ( 'NONE', *, *, #38622, .T. ) ;
#44484=EDGE_LOOP ( 'NONE', ( #41540, #20814, #21181, #21379, #21384 ) ) ;
#44494=VERTEX_POINT ( 'NONE', #16985 ) ;
#44499=VERTEX_POINT ( 'NONE', #30877 ) ;
#44514=DIRECTION ( 'NONE',  ( -0.2768435750659241079, -0.3568721902840695792, 0.8921882507333129819 ) ) ;
#44578=EDGE_CURVE ( 'NONE', #35636, #42996, #12149, .T. ) ;
#44579=EDGE_CURVE ( 'NONE', #32876, #36279, #29247, .T. ) ;
#44597=AXIS2_PLACEMENT_3D ( 'NONE', #35526, #27600, #41514 ) ;
#44623=ORIENTED_EDGE ( 'NONE', *, *, #17533, .F. ) ;
#44629=VECTOR ( 'NONE', #12084, 1000.000000000000227 ) ;
#44641=ORIENTED_EDGE ( 'NONE', *, *, #23727, .F. ) ;
#44676=ORIENTED_EDGE ( 'NONE', *, *, #14805, .F. ) ;
#44682=VERTEX_POINT ( 'NONE', #38745 ) ;
#44706=FACE_OUTER_BOUND ( 'NONE', #33531, .T. ) ;
#44742=LINE ( 'NONE', #10089, #21450 ) ;
#44755=CARTESIAN_POINT ( 'NONE',  ( 68.89072742534011695, -72.29603325525536661, -37.25697179492874511 ) ) ;
#44789=EDGE_LOOP ( 'NONE', ( #43312, #37234, #5579, #7357, #23524 ) ) ;
#44794=VERTEX_POINT ( 'NONE', #21879 ) ;
#44797=CIRCLE ( 'NONE', #29478, 2.999999999999999556 ) ;
#44804=DIRECTION ( 'NONE',  ( -0.2768435750659243300, -0.3568721902840689131, 0.8921882507333129819 ) ) ;
#44837=CIRCLE ( 'NONE', #12042, 2.999999999999999556 ) ;
#44915=DIRECTION ( 'NONE',  ( -0.000000000000000000, -0.9284778069183720062, -0.3713878862591650232 ) ) ;
#44917=PLANE ( 'NONE',  #12140 ) ;
#44930=CARTESIAN_POINT ( 'NONE',  ( 72.54180985774836188, -53.22909301380743585, -33.76528779565084903 ) ) ;
#44946=CARTESIAN_POINT ( 'NONE',  ( 70.19189222814998175, -60.76597359474132531, -37.50918677187066663 ) ) ;
#44966=DIRECTION ( 'NONE',  ( 0.2397535688815952137, -0.1551785207689905521, -0.9583516332226319490 ) ) ;
#45004=ORIENTED_EDGE ( 'NONE', *, *, #30653, .F. ) ;
#45014=VECTOR ( 'NONE', #18823, 1000.000000000000114 ) ;
#45046=CIRCLE ( 'NONE', #7887, 2.445500000000004448 ) ;
#45051=CARTESIAN_POINT ( 'NONE',  ( 73.07463722459043254, -57.36051141757233296, -35.25250588052404765 ) ) ;
#45101=ORIENTED_EDGE ( 'NONE', *, *, #3140, .T. ) ;
#45103=ORIENTED_EDGE ( 'NONE', *, *, #36564, .T. ) ;
#45119=DIRECTION ( 'NONE',  ( -0.000000000000000000, -0.9284778069183718952, -0.3713878862591649677 ) ) ;
#45138=EDGE_CURVE ( 'NONE', #23460, #32855, #31735, .T. ) ;
#45145=DIRECTION ( 'NONE',  ( 0.000000000000000000, 0.9284778069183720062, 0.3713878862591650232 ) ) ;
#45184=COLOUR_RGB('Black',0.12,0.14,0.17);
#45185=FILL_AREA_STYLE_COLOUR('',#45184);
#45186=FILL_AREA_STYLE('',(#45185));
#45187=SURFACE_STYLE_FILL_AREA(#45186);
#45188=SURFACE_SIDE_STYLE('',(#45187));
#45189=SURFACE_STYLE_USAGE(.BOTH.,#45188);
#45190=PRESENTATION_STYLE_ASSIGNMENT((#45189));
ENDSEC;
END-ISO-10303-21;
